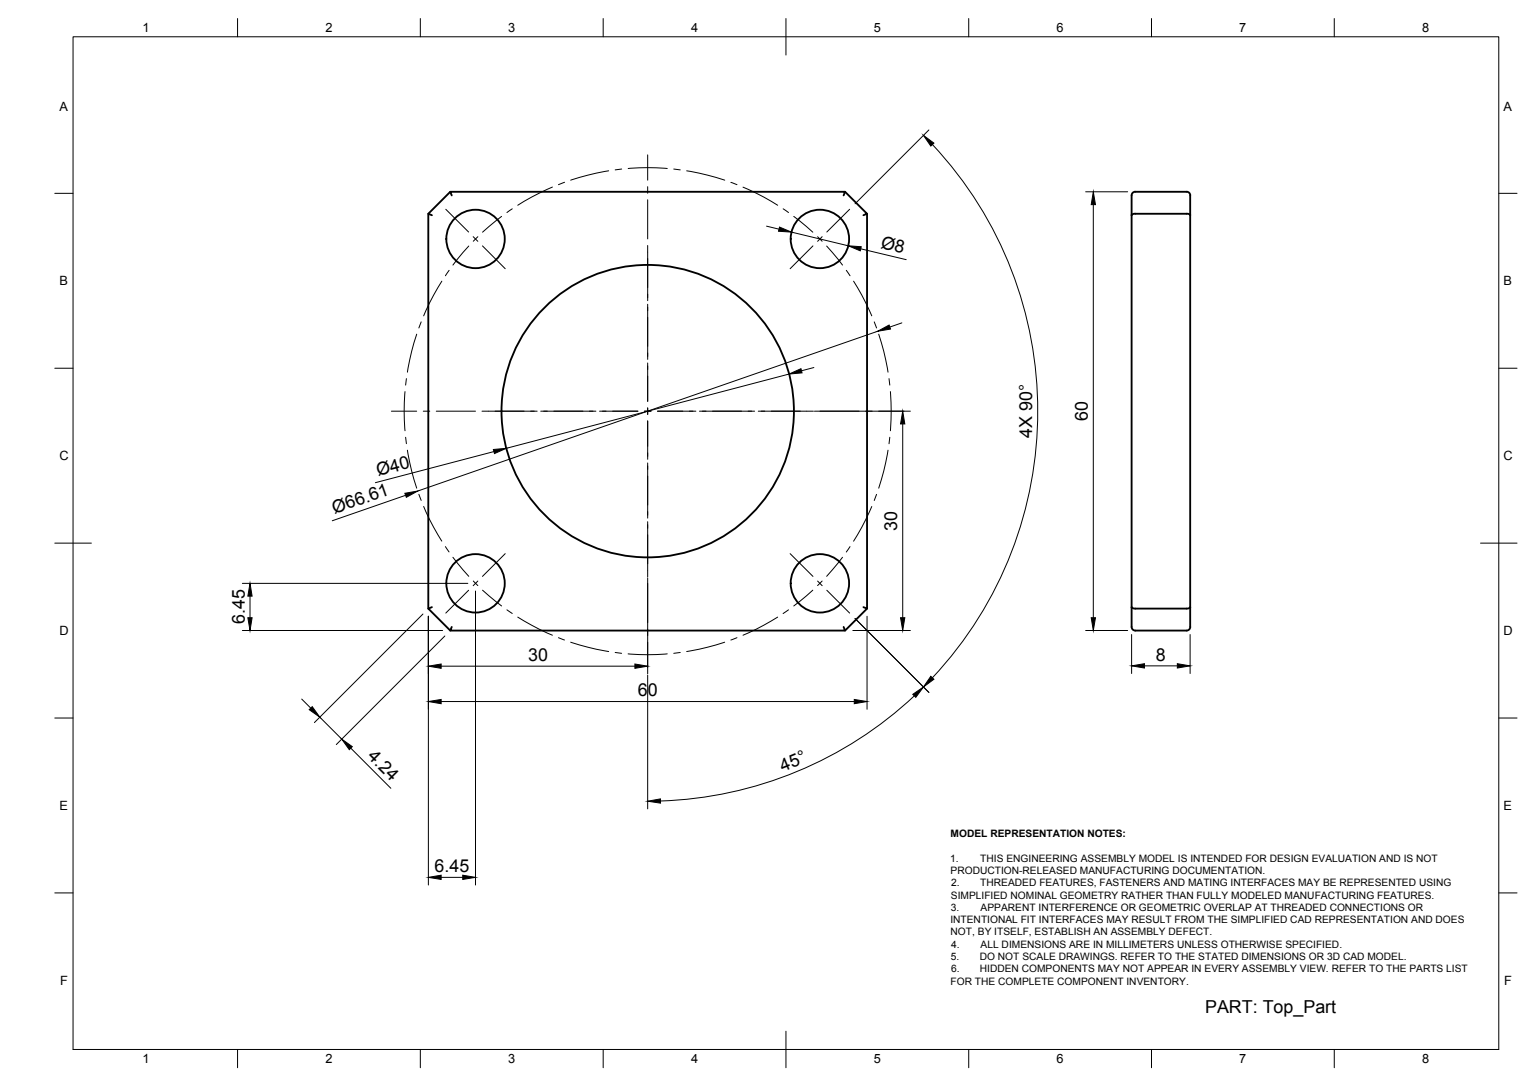
ISO-10303-21;
HEADER;
/* Generated by software containing ST-Developer
 * from STEP Tools, Inc. (www.steptools.com) 
 */

FILE_DESCRIPTION(
/* description */ (''),
/* implementation_level */ '2;1');

FILE_NAME(
/* name */ 'Top_Part.step',
/* time_stamp */ '2026-10-05T14:32:37-07:00',
/* author */ (''),
/* organization */ (''),
/* preprocessor_version */ 'ST-DEVELOPER v20.2',
/* originating_system */ 'Autodesk Translation Framework v15.15.0.0',
/* authorisation */ '');

FILE_SCHEMA (('AUTOMOTIVE_DESIGN { 1 0 10303 214 3 1 1 }'));
ENDSEC;

DATA;
#10=MECHANICAL_DESIGN_GEOMETRIC_PRESENTATION_REPRESENTATION('',(#494),#74103);
#486=SHAPE_REPRESENTATION_RELATIONSHIP('SRR','None',#74128,#490);
#490=ADVANCED_BREP_SHAPE_REPRESENTATION('',(#498),#74099);
#494=STYLED_ITEM('',(#74157),#498);
#498=MANIFOLD_SOLID_BREP('Body1',#4573);
#502=TOROIDAL_SURFACE('',#4660,4.5,0.5);
#503=TOROIDAL_SURFACE('',#4667,4.5,0.5);
#504=TOROIDAL_SURFACE('',#4674,4.5,0.5);
#505=TOROIDAL_SURFACE('',#4681,20.5,0.5);
#506=TOROIDAL_SURFACE('',#4686,4.5,0.5);
#507=TOROIDAL_SURFACE('',#4716,4.5,0.5);
#508=TOROIDAL_SURFACE('',#4718,4.5,0.5);
#509=TOROIDAL_SURFACE('',#4720,4.5,0.5);
#510=TOROIDAL_SURFACE('',#4722,20.5,0.5);
#511=TOROIDAL_SURFACE('',#4724,4.5,0.5);
#526=ELLIPSE('',#4635,0.541196100146199,0.5);
#527=ELLIPSE('',#4636,0.541196100146197,0.5);
#528=ELLIPSE('',#4638,0.541196100146197,0.5);
#529=ELLIPSE('',#4640,0.541196100146199,0.5);
#530=ELLIPSE('',#4642,0.541196100146199,0.5);
#531=ELLIPSE('',#4643,0.541196100146197,0.5);
#532=ELLIPSE('',#4645,0.541196100146197,0.5);
#533=ELLIPSE('',#4648,0.541196100146199,0.5);
#534=ELLIPSE('',#4694,0.541196100146197,0.5);
#535=ELLIPSE('',#4695,0.541196100146197,0.5);
#536=ELLIPSE('',#4697,0.541196100146197,0.5);
#537=ELLIPSE('',#4699,0.541196100146197,0.5);
#538=ELLIPSE('',#4701,0.541196100146197,0.5);
#539=ELLIPSE('',#4703,0.541196100146197,0.5);
#540=ELLIPSE('',#4705,0.541196100146197,0.5);
#541=ELLIPSE('',#4707,0.541196100146197,0.5);
#558=FACE_BOUND('',#800,.T.);
#559=FACE_BOUND('',#802,.T.);
#560=FACE_BOUND('',#817,.T.);
#561=FACE_BOUND('',#818,.T.);
#562=FACE_BOUND('',#819,.T.);
#563=FACE_BOUND('',#820,.T.);
#564=FACE_BOUND('',#821,.T.);
#565=FACE_BOUND('',#842,.T.);
#566=FACE_BOUND('',#843,.T.);
#567=FACE_BOUND('',#844,.T.);
#568=FACE_BOUND('',#845,.T.);
#569=FACE_BOUND('',#846,.T.);
#584=PLANE('',#4627);
#585=PLANE('',#4629);
#586=PLANE('',#4650);
#587=PLANE('',#4651);
#588=PLANE('',#4652);
#589=PLANE('',#4653);
#590=PLANE('',#4654);
#591=PLANE('',#4709);
#592=PLANE('',#4710);
#593=PLANE('',#4726);
#594=PLANE('',#4727);
#595=PLANE('',#4728);
#612=FACE_OUTER_BOUND('',#798,.T.);
#613=FACE_OUTER_BOUND('',#799,.T.);
#614=FACE_OUTER_BOUND('',#801,.T.);
#615=FACE_OUTER_BOUND('',#803,.T.);
#616=FACE_OUTER_BOUND('',#804,.T.);
#617=FACE_OUTER_BOUND('',#805,.T.);
#618=FACE_OUTER_BOUND('',#806,.T.);
#619=FACE_OUTER_BOUND('',#807,.T.);
#620=FACE_OUTER_BOUND('',#808,.T.);
#621=FACE_OUTER_BOUND('',#809,.T.);
#622=FACE_OUTER_BOUND('',#810,.T.);
#623=FACE_OUTER_BOUND('',#811,.T.);
#624=FACE_OUTER_BOUND('',#812,.T.);
#625=FACE_OUTER_BOUND('',#813,.T.);
#626=FACE_OUTER_BOUND('',#814,.T.);
#627=FACE_OUTER_BOUND('',#815,.T.);
#628=FACE_OUTER_BOUND('',#816,.T.);
#629=FACE_OUTER_BOUND('',#822,.T.);
#630=FACE_OUTER_BOUND('',#823,.T.);
#631=FACE_OUTER_BOUND('',#824,.T.);
#632=FACE_OUTER_BOUND('',#825,.T.);
#633=FACE_OUTER_BOUND('',#826,.T.);
#634=FACE_OUTER_BOUND('',#827,.T.);
#635=FACE_OUTER_BOUND('',#828,.T.);
#636=FACE_OUTER_BOUND('',#829,.T.);
#637=FACE_OUTER_BOUND('',#830,.T.);
#638=FACE_OUTER_BOUND('',#831,.T.);
#639=FACE_OUTER_BOUND('',#832,.T.);
#640=FACE_OUTER_BOUND('',#833,.T.);
#641=FACE_OUTER_BOUND('',#834,.T.);
#642=FACE_OUTER_BOUND('',#835,.T.);
#643=FACE_OUTER_BOUND('',#836,.T.);
#644=FACE_OUTER_BOUND('',#837,.T.);
#645=FACE_OUTER_BOUND('',#838,.T.);
#646=FACE_OUTER_BOUND('',#839,.T.);
#647=FACE_OUTER_BOUND('',#840,.T.);
#648=FACE_OUTER_BOUND('',#841,.T.);
#649=FACE_OUTER_BOUND('',#847,.T.);
#650=FACE_OUTER_BOUND('',#848,.T.);
#651=FACE_OUTER_BOUND('',#849,.T.);
#652=FACE_OUTER_BOUND('',#850,.T.);
#653=FACE_OUTER_BOUND('',#851,.T.);
#654=FACE_OUTER_BOUND('',#852,.T.);
#655=FACE_OUTER_BOUND('',#853,.T.);
#656=FACE_OUTER_BOUND('',#854,.T.);
#798=EDGE_LOOP('',(#2771,#2772,#2773,#2774));
#799=EDGE_LOOP('',(#2775));
#800=EDGE_LOOP('',(#2776));
#801=EDGE_LOOP('',(#2777));
#802=EDGE_LOOP('',(#2778));
#803=EDGE_LOOP('',(#2779,#2780,#2781,#2782,#2783));
#804=EDGE_LOOP('',(#2784,#2785,#2786,#2787));
#805=EDGE_LOOP('',(#2788,#2789,#2790,#2791));
#806=EDGE_LOOP('',(#2792,#2793,#2794,#2795));
#807=EDGE_LOOP('',(#2796,#2797,#2798,#2799));
#808=EDGE_LOOP('',(#2800,#2801,#2802,#2803));
#809=EDGE_LOOP('',(#2804,#2805,#2806,#2807));
#810=EDGE_LOOP('',(#2808,#2809,#2810,#2811));
#811=EDGE_LOOP('',(#2812,#2813,#2814,#2815));
#812=EDGE_LOOP('',(#2816,#2817,#2818,#2819));
#813=EDGE_LOOP('',(#2820,#2821,#2822,#2823));
#814=EDGE_LOOP('',(#2824,#2825,#2826,#2827));
#815=EDGE_LOOP('',(#2828,#2829,#2830,#2831));
#816=EDGE_LOOP('',(#2832,#2833,#2834,#2835,#2836,#2837,#2838,#2839));
#817=EDGE_LOOP('',(#2840));
#818=EDGE_LOOP('',(#2841));
#819=EDGE_LOOP('',(#2842));
#820=EDGE_LOOP('',(#2843));
#821=EDGE_LOOP('',(#2844));
#822=EDGE_LOOP('',(#2845,#2846,#2847,#2848,#2849));
#823=EDGE_LOOP('',(#2850,#2851,#2852,#2853,#2854,#2855));
#824=EDGE_LOOP('',(#2856,#2857,#2858,#2859,#2860));
#825=EDGE_LOOP('',(#2861,#2862,#2863,#2864,#2865,#2866));
#826=EDGE_LOOP('',(#2867,#2868,#2869,#2870,#2871));
#827=EDGE_LOOP('',(#2872,#2873,#2874,#2875,#2876,#2877));
#828=EDGE_LOOP('',(#2878,#2879,#2880,#2881,#2882));
#829=EDGE_LOOP('',(#2883,#2884,#2885,#2886,#2887));
#830=EDGE_LOOP('',(#2888,#2889,#2890,#2891,#2892));
#831=EDGE_LOOP('',(#2893,#2894,#2895,#2896,#2897,#2898));
#832=EDGE_LOOP('',(#2899,#2900,#2901,#2902));
#833=EDGE_LOOP('',(#2903,#2904,#2905,#2906));
#834=EDGE_LOOP('',(#2907,#2908,#2909,#2910));
#835=EDGE_LOOP('',(#2911,#2912,#2913,#2914));
#836=EDGE_LOOP('',(#2915,#2916,#2917,#2918));
#837=EDGE_LOOP('',(#2919,#2920,#2921,#2922));
#838=EDGE_LOOP('',(#2923,#2924,#2925,#2926));
#839=EDGE_LOOP('',(#2927,#2928,#2929,#2930));
#840=EDGE_LOOP('',(#2931,#2932,#2933,#2934));
#841=EDGE_LOOP('',(#2935,#2936,#2937,#2938,#2939,#2940,#2941,#2942));
#842=EDGE_LOOP('',(#2943));
#843=EDGE_LOOP('',(#2944));
#844=EDGE_LOOP('',(#2945));
#845=EDGE_LOOP('',(#2946));
#846=EDGE_LOOP('',(#2947));
#847=EDGE_LOOP('',(#2948,#2949,#2950,#2951,#2952));
#848=EDGE_LOOP('',(#2953,#2954,#2955,#2956,#2957));
#849=EDGE_LOOP('',(#2958,#2959,#2960,#2961,#2962));
#850=EDGE_LOOP('',(#2963,#2964,#2965,#2966,#2967));
#851=EDGE_LOOP('',(#2968,#2969,#2970,#2971,#2972));
#852=EDGE_LOOP('',(#2973,#2974,#2975,#2976));
#853=EDGE_LOOP('',(#2977,#2978,#2979,#2980));
#854=EDGE_LOOP('',(#2981,#2982,#2983,#2984));
#1010=LINE('',#5781,#1188);
#1011=LINE('',#5794,#1189);
#1012=LINE('',#5798,#1190);
#1013=LINE('',#5802,#1191);
#1014=LINE('',#5806,#1192);
#1015=LINE('',#5809,#1193);
#1016=LINE('',#5812,#1194);
#1017=LINE('',#5815,#1195);
#1018=LINE('',#5819,#1196);
#1019=LINE('',#5823,#1197);
#1020=LINE('',#5827,#1198);
#1021=LINE('',#5829,#1199);
#1022=LINE('',#5832,#1200);
#1023=LINE('',#5833,#1201);
#1024=LINE('',#5836,#1202);
#1025=LINE('',#5838,#1203);
#1026=LINE('',#5841,#1204);
#1027=LINE('',#5842,#1205);
#1028=LINE('',#5845,#1206);
#1029=LINE('',#5847,#1207);
#1030=LINE('',#5848,#1208);
#1031=LINE('',#5851,#1209);
#1032=LINE('',#5852,#1210);
#1033=LINE('',#5855,#1211);
#1034=LINE('',#5856,#1212);
#1035=LINE('',#5859,#1213);
#1036=LINE('',#5860,#1214);
#1037=LINE('',#5880,#1215);
#1038=LINE('',#5892,#1216);
#1039=LINE('',#5904,#1217);
#1040=LINE('',#5912,#1218);
#1041=LINE('',#5924,#1219);
#1042=LINE('',#5931,#1220);
#1043=LINE('',#5934,#1221);
#1044=LINE('',#5938,#1222);
#1045=LINE('',#5941,#1223);
#1046=LINE('',#5944,#1224);
#1047=LINE('',#5947,#1225);
#1048=LINE('',#5950,#1226);
#1049=LINE('',#5952,#1227);
#1050=LINE('',#5955,#1228);
#1051=LINE('',#5959,#1229);
#1052=LINE('',#5963,#1230);
#1053=LINE('',#5966,#1231);
#1054=LINE('',#5968,#1232);
#1055=LINE('',#5991,#1233);
#1056=LINE('',#5993,#1234);
#1188=VECTOR('',#4955,20.5);
#1189=VECTOR('',#4972,20.);
#1190=VECTOR('',#4975,10.);
#1191=VECTOR('',#4978,10.);
#1192=VECTOR('',#4983,10.);
#1193=VECTOR('',#4986,9.99999999999999);
#1194=VECTOR('',#4989,10.);
#1195=VECTOR('',#4992,10.);
#1196=VECTOR('',#4995,10.);
#1197=VECTOR('',#4998,10.);
#1198=VECTOR('',#5003,9.99999999999999);
#1199=VECTOR('',#5004,10.);
#1200=VECTOR('',#5009,10.);
#1201=VECTOR('',#5010,9.99999999999999);
#1202=VECTOR('',#5013,10.);
#1203=VECTOR('',#5014,10.);
#1204=VECTOR('',#5019,9.99999999999999);
#1205=VECTOR('',#5020,10.);
#1206=VECTOR('',#5023,10.);
#1207=VECTOR('',#5024,9.99999999999999);
#1208=VECTOR('',#5025,10.);
#1209=VECTOR('',#5028,10.);
#1210=VECTOR('',#5029,10.);
#1211=VECTOR('',#5032,10.);
#1212=VECTOR('',#5033,9.99999999999999);
#1213=VECTOR('',#5036,10.);
#1214=VECTOR('',#5037,10.);
#1215=VECTOR('',#5060,4.);
#1216=VECTOR('',#5075,4.);
#1217=VECTOR('',#5090,4.);
#1218=VECTOR('',#5101,20.);
#1219=VECTOR('',#5116,4.);
#1220=VECTOR('',#5123,10.);
#1221=VECTOR('',#5126,10.);
#1222=VECTOR('',#5131,10.);
#1223=VECTOR('',#5134,9.99999999999999);
#1224=VECTOR('',#5137,10.);
#1225=VECTOR('',#5140,10.);
#1226=VECTOR('',#5143,10.);
#1227=VECTOR('',#5146,9.99999999999999);
#1228=VECTOR('',#5149,10.);
#1229=VECTOR('',#5154,10.);
#1230=VECTOR('',#5159,10.);
#1231=VECTOR('',#5164,10.);
#1232=VECTOR('',#5167,10.);
#1233=VECTOR('',#5202,10.);
#1234=VECTOR('',#5205,10.);
#1366=CIRCLE('',#4625,20.5);
#1367=CIRCLE('',#4626,20.5);
#1368=CIRCLE('',#4628,20.);
#1369=CIRCLE('',#4630,20.);
#1370=CIRCLE('',#4632,20.);
#1371=CIRCLE('',#4633,20.);
#1372=CIRCLE('',#4655,4.5);
#1373=CIRCLE('',#4656,4.5);
#1374=CIRCLE('',#4657,4.5);
#1375=CIRCLE('',#4658,20.5);
#1376=CIRCLE('',#4659,4.5);
#1377=CIRCLE('',#4661,4.);
#1378=CIRCLE('',#4662,0.5);
#1379=CIRCLE('',#4663,4.);
#1380=CIRCLE('',#4665,4.);
#1381=CIRCLE('',#4666,4.);
#1382=CIRCLE('',#4668,4.);
#1383=CIRCLE('',#4669,0.5);
#1384=CIRCLE('',#4670,4.);
#1385=CIRCLE('',#4672,4.);
#1386=CIRCLE('',#4673,4.);
#1387=CIRCLE('',#4675,4.);
#1388=CIRCLE('',#4676,0.5);
#1389=CIRCLE('',#4677,4.);
#1390=CIRCLE('',#4679,4.);
#1391=CIRCLE('',#4680,4.);
#1392=CIRCLE('',#4682,0.5);
#1393=CIRCLE('',#4684,20.);
#1394=CIRCLE('',#4685,20.);
#1395=CIRCLE('',#4687,4.);
#1396=CIRCLE('',#4688,0.5);
#1397=CIRCLE('',#4689,4.);
#1398=CIRCLE('',#4691,4.);
#1399=CIRCLE('',#4692,4.);
#1400=CIRCLE('',#4711,4.5);
#1401=CIRCLE('',#4712,4.5);
#1402=CIRCLE('',#4713,4.5);
#1403=CIRCLE('',#4714,20.5);
#1404=CIRCLE('',#4715,4.5);
#1405=CIRCLE('',#4717,0.5);
#1406=CIRCLE('',#4719,0.5);
#1407=CIRCLE('',#4721,0.5);
#1408=CIRCLE('',#4723,0.5);
#1409=CIRCLE('',#4725,0.5);
#1461=VERTEX_POINT('',#5778);
#1462=VERTEX_POINT('',#5780);
#1463=VERTEX_POINT('',#5784);
#1464=VERTEX_POINT('',#5787);
#1465=VERTEX_POINT('',#5790);
#1466=VERTEX_POINT('',#5791);
#1467=VERTEX_POINT('',#5796);
#1468=VERTEX_POINT('',#5797);
#1469=VERTEX_POINT('',#5799);
#1470=VERTEX_POINT('',#5801);
#1471=VERTEX_POINT('',#5805);
#1472=VERTEX_POINT('',#5807);
#1473=VERTEX_POINT('',#5811);
#1474=VERTEX_POINT('',#5813);
#1475=VERTEX_POINT('',#5817);
#1476=VERTEX_POINT('',#5818);
#1477=VERTEX_POINT('',#5820);
#1478=VERTEX_POINT('',#5822);
#1479=VERTEX_POINT('',#5826);
#1480=VERTEX_POINT('',#5828);
#1481=VERTEX_POINT('',#5835);
#1482=VERTEX_POINT('',#5837);
#1483=VERTEX_POINT('',#5844);
#1484=VERTEX_POINT('',#5846);
#1485=VERTEX_POINT('',#5850);
#1486=VERTEX_POINT('',#5854);
#1487=VERTEX_POINT('',#5858);
#1488=VERTEX_POINT('',#5862);
#1489=VERTEX_POINT('',#5864);
#1490=VERTEX_POINT('',#5866);
#1491=VERTEX_POINT('',#5868);
#1492=VERTEX_POINT('',#5870);
#1493=VERTEX_POINT('',#5873);
#1494=VERTEX_POINT('',#5874);
#1495=VERTEX_POINT('',#5879);
#1496=VERTEX_POINT('',#5881);
#1497=VERTEX_POINT('',#5885);
#1498=VERTEX_POINT('',#5886);
#1499=VERTEX_POINT('',#5891);
#1500=VERTEX_POINT('',#5893);
#1501=VERTEX_POINT('',#5897);
#1502=VERTEX_POINT('',#5898);
#1503=VERTEX_POINT('',#5903);
#1504=VERTEX_POINT('',#5905);
#1505=VERTEX_POINT('',#5911);
#1506=VERTEX_POINT('',#5913);
#1507=VERTEX_POINT('',#5917);
#1508=VERTEX_POINT('',#5918);
#1509=VERTEX_POINT('',#5923);
#1510=VERTEX_POINT('',#5925);
#1511=VERTEX_POINT('',#5929);
#1512=VERTEX_POINT('',#5930);
#1513=VERTEX_POINT('',#5932);
#1514=VERTEX_POINT('',#5937);
#1515=VERTEX_POINT('',#5939);
#1516=VERTEX_POINT('',#5943);
#1517=VERTEX_POINT('',#5945);
#1518=VERTEX_POINT('',#5949);
#1519=VERTEX_POINT('',#5954);
#1520=VERTEX_POINT('',#5958);
#1521=VERTEX_POINT('',#5962);
#1522=VERTEX_POINT('',#5970);
#1523=VERTEX_POINT('',#5972);
#1524=VERTEX_POINT('',#5974);
#1525=VERTEX_POINT('',#5976);
#1526=VERTEX_POINT('',#5978);
#2029=EDGE_CURVE('',#1461,#1461,#1366,.T.);
#2030=EDGE_CURVE('',#1461,#1462,#1010,.T.);
#2031=EDGE_CURVE('',#1462,#1462,#1367,.T.);
#2032=EDGE_CURVE('',#1463,#1463,#1368,.T.);
#2033=EDGE_CURVE('',#1464,#1464,#1369,.T.);
#2034=EDGE_CURVE('',#1465,#1466,#1370,.T.);
#2035=EDGE_CURVE('',#1466,#1465,#1371,.T.);
#2036=EDGE_CURVE('',#1466,#1464,#1011,.T.);
#2037=EDGE_CURVE('',#1467,#1468,#1012,.T.);
#2038=EDGE_CURVE('',#1468,#1469,#526,.T.);
#2039=EDGE_CURVE('',#1469,#1470,#1013,.T.);
#2040=EDGE_CURVE('',#1467,#1470,#527,.T.);
#2041=EDGE_CURVE('',#1468,#1471,#1014,.T.);
#2042=EDGE_CURVE('',#1471,#1472,#528,.T.);
#2043=EDGE_CURVE('',#1472,#1469,#1015,.T.);
#2044=EDGE_CURVE('',#1471,#1473,#1016,.T.);
#2045=EDGE_CURVE('',#1473,#1474,#529,.T.);
#2046=EDGE_CURVE('',#1474,#1472,#1017,.T.);
#2047=EDGE_CURVE('',#1475,#1476,#1018,.T.);
#2048=EDGE_CURVE('',#1476,#1477,#530,.T.);
#2049=EDGE_CURVE('',#1477,#1478,#1019,.T.);
#2050=EDGE_CURVE('',#1478,#1475,#531,.T.);
#2051=EDGE_CURVE('',#1479,#1477,#1020,.T.);
#2052=EDGE_CURVE('',#1476,#1480,#1021,.T.);
#2053=EDGE_CURVE('',#1480,#1479,#532,.T.);
#2054=EDGE_CURVE('',#1473,#1475,#1022,.T.);
#2055=EDGE_CURVE('',#1478,#1474,#1023,.T.);
#2056=EDGE_CURVE('',#1481,#1479,#1024,.T.);
#2057=EDGE_CURVE('',#1480,#1482,#1025,.T.);
#2058=EDGE_CURVE('',#1482,#1481,#533,.T.);
#2059=EDGE_CURVE('',#1470,#1481,#1026,.T.);
#2060=EDGE_CURVE('',#1482,#1467,#1027,.T.);
#2061=EDGE_CURVE('',#1472,#1483,#1028,.T.);
#2062=EDGE_CURVE('',#1484,#1483,#1029,.T.);
#2063=EDGE_CURVE('',#1469,#1484,#1030,.T.);
#2064=EDGE_CURVE('',#1474,#1485,#1031,.T.);
#2065=EDGE_CURVE('',#1483,#1485,#1032,.T.);
#2066=EDGE_CURVE('',#1478,#1486,#1033,.T.);
#2067=EDGE_CURVE('',#1485,#1486,#1034,.T.);
#2068=EDGE_CURVE('',#1477,#1487,#1035,.T.);
#2069=EDGE_CURVE('',#1486,#1487,#1036,.T.);
#2070=EDGE_CURVE('',#1488,#1488,#1372,.T.);
#2071=EDGE_CURVE('',#1489,#1489,#1373,.T.);
#2072=EDGE_CURVE('',#1490,#1490,#1374,.T.);
#2073=EDGE_CURVE('',#1491,#1491,#1375,.T.);
#2074=EDGE_CURVE('',#1492,#1492,#1376,.T.);
#2075=EDGE_CURVE('',#1493,#1494,#1377,.T.);
#2076=EDGE_CURVE('',#1494,#1488,#1378,.T.);
#2077=EDGE_CURVE('',#1494,#1493,#1379,.T.);
#2078=EDGE_CURVE('',#1493,#1495,#1037,.T.);
#2079=EDGE_CURVE('',#1496,#1495,#1380,.T.);
#2080=EDGE_CURVE('',#1495,#1496,#1381,.T.);
#2081=EDGE_CURVE('',#1497,#1498,#1382,.T.);
#2082=EDGE_CURVE('',#1498,#1492,#1383,.T.);
#2083=EDGE_CURVE('',#1498,#1497,#1384,.T.);
#2084=EDGE_CURVE('',#1497,#1499,#1038,.T.);
#2085=EDGE_CURVE('',#1500,#1499,#1385,.T.);
#2086=EDGE_CURVE('',#1499,#1500,#1386,.T.);
#2087=EDGE_CURVE('',#1501,#1502,#1387,.T.);
#2088=EDGE_CURVE('',#1502,#1489,#1388,.T.);
#2089=EDGE_CURVE('',#1502,#1501,#1389,.T.);
#2090=EDGE_CURVE('',#1501,#1503,#1039,.T.);
#2091=EDGE_CURVE('',#1504,#1503,#1390,.T.);
#2092=EDGE_CURVE('',#1503,#1504,#1391,.T.);
#2093=EDGE_CURVE('',#1465,#1491,#1392,.T.);
#2094=EDGE_CURVE('',#1463,#1505,#1040,.T.);
#2095=EDGE_CURVE('',#1506,#1505,#1393,.T.);
#2096=EDGE_CURVE('',#1505,#1506,#1394,.T.);
#2097=EDGE_CURVE('',#1507,#1508,#1395,.T.);
#2098=EDGE_CURVE('',#1508,#1490,#1396,.T.);
#2099=EDGE_CURVE('',#1508,#1507,#1397,.T.);
#2100=EDGE_CURVE('',#1507,#1509,#1041,.T.);
#2101=EDGE_CURVE('',#1510,#1509,#1398,.T.);
#2102=EDGE_CURVE('',#1509,#1510,#1399,.T.);
#2103=EDGE_CURVE('',#1511,#1512,#1042,.T.);
#2104=EDGE_CURVE('',#1512,#1513,#534,.T.);
#2105=EDGE_CURVE('',#1513,#1484,#1043,.T.);
#2106=EDGE_CURVE('',#1511,#1484,#535,.T.);
#2107=EDGE_CURVE('',#1512,#1514,#1044,.T.);
#2108=EDGE_CURVE('',#1514,#1515,#536,.T.);
#2109=EDGE_CURVE('',#1515,#1513,#1045,.T.);
#2110=EDGE_CURVE('',#1514,#1516,#1046,.T.);
#2111=EDGE_CURVE('',#1516,#1517,#537,.T.);
#2112=EDGE_CURVE('',#1517,#1515,#1047,.T.);
#2113=EDGE_CURVE('',#1516,#1518,#1048,.T.);
#2114=EDGE_CURVE('',#1518,#1487,#538,.T.);
#2115=EDGE_CURVE('',#1487,#1517,#1049,.T.);
#2116=EDGE_CURVE('',#1518,#1519,#1050,.T.);
#2117=EDGE_CURVE('',#1519,#1486,#539,.T.);
#2118=EDGE_CURVE('',#1519,#1520,#1051,.T.);
#2119=EDGE_CURVE('',#1520,#1485,#540,.T.);
#2120=EDGE_CURVE('',#1520,#1521,#1052,.T.);
#2121=EDGE_CURVE('',#1521,#1483,#541,.T.);
#2122=EDGE_CURVE('',#1521,#1511,#1053,.T.);
#2123=EDGE_CURVE('',#1470,#1513,#1054,.T.);
#2124=EDGE_CURVE('',#1522,#1522,#1400,.T.);
#2125=EDGE_CURVE('',#1523,#1523,#1401,.T.);
#2126=EDGE_CURVE('',#1524,#1524,#1402,.T.);
#2127=EDGE_CURVE('',#1525,#1525,#1403,.T.);
#2128=EDGE_CURVE('',#1526,#1526,#1404,.T.);
#2129=EDGE_CURVE('',#1522,#1496,#1405,.T.);
#2130=EDGE_CURVE('',#1526,#1500,#1406,.T.);
#2131=EDGE_CURVE('',#1523,#1504,#1407,.T.);
#2132=EDGE_CURVE('',#1525,#1506,#1408,.T.);
#2133=EDGE_CURVE('',#1524,#1510,#1409,.T.);
#2134=EDGE_CURVE('',#1481,#1515,#1055,.T.);
#2135=EDGE_CURVE('',#1479,#1517,#1056,.T.);
#2771=ORIENTED_EDGE('',*,*,#2029,.F.);
#2772=ORIENTED_EDGE('',*,*,#2030,.T.);
#2773=ORIENTED_EDGE('',*,*,#2031,.T.);
#2774=ORIENTED_EDGE('',*,*,#2030,.F.);
#2775=ORIENTED_EDGE('',*,*,#2031,.F.);
#2776=ORIENTED_EDGE('',*,*,#2032,.F.);
#2777=ORIENTED_EDGE('',*,*,#2029,.T.);
#2778=ORIENTED_EDGE('',*,*,#2033,.F.);
#2779=ORIENTED_EDGE('',*,*,#2034,.F.);
#2780=ORIENTED_EDGE('',*,*,#2035,.F.);
#2781=ORIENTED_EDGE('',*,*,#2036,.T.);
#2782=ORIENTED_EDGE('',*,*,#2033,.T.);
#2783=ORIENTED_EDGE('',*,*,#2036,.F.);
#2784=ORIENTED_EDGE('',*,*,#2037,.T.);
#2785=ORIENTED_EDGE('',*,*,#2038,.T.);
#2786=ORIENTED_EDGE('',*,*,#2039,.T.);
#2787=ORIENTED_EDGE('',*,*,#2040,.F.);
#2788=ORIENTED_EDGE('',*,*,#2041,.T.);
#2789=ORIENTED_EDGE('',*,*,#2042,.T.);
#2790=ORIENTED_EDGE('',*,*,#2043,.T.);
#2791=ORIENTED_EDGE('',*,*,#2038,.F.);
#2792=ORIENTED_EDGE('',*,*,#2044,.T.);
#2793=ORIENTED_EDGE('',*,*,#2045,.T.);
#2794=ORIENTED_EDGE('',*,*,#2046,.T.);
#2795=ORIENTED_EDGE('',*,*,#2042,.F.);
#2796=ORIENTED_EDGE('',*,*,#2047,.T.);
#2797=ORIENTED_EDGE('',*,*,#2048,.T.);
#2798=ORIENTED_EDGE('',*,*,#2049,.T.);
#2799=ORIENTED_EDGE('',*,*,#2050,.T.);
#2800=ORIENTED_EDGE('',*,*,#2051,.T.);
#2801=ORIENTED_EDGE('',*,*,#2048,.F.);
#2802=ORIENTED_EDGE('',*,*,#2052,.T.);
#2803=ORIENTED_EDGE('',*,*,#2053,.T.);
#2804=ORIENTED_EDGE('',*,*,#2054,.T.);
#2805=ORIENTED_EDGE('',*,*,#2050,.F.);
#2806=ORIENTED_EDGE('',*,*,#2055,.T.);
#2807=ORIENTED_EDGE('',*,*,#2045,.F.);
#2808=ORIENTED_EDGE('',*,*,#2056,.T.);
#2809=ORIENTED_EDGE('',*,*,#2053,.F.);
#2810=ORIENTED_EDGE('',*,*,#2057,.T.);
#2811=ORIENTED_EDGE('',*,*,#2058,.T.);
#2812=ORIENTED_EDGE('',*,*,#2059,.T.);
#2813=ORIENTED_EDGE('',*,*,#2058,.F.);
#2814=ORIENTED_EDGE('',*,*,#2060,.T.);
#2815=ORIENTED_EDGE('',*,*,#2040,.T.);
#2816=ORIENTED_EDGE('',*,*,#2043,.F.);
#2817=ORIENTED_EDGE('',*,*,#2061,.T.);
#2818=ORIENTED_EDGE('',*,*,#2062,.F.);
#2819=ORIENTED_EDGE('',*,*,#2063,.F.);
#2820=ORIENTED_EDGE('',*,*,#2046,.F.);
#2821=ORIENTED_EDGE('',*,*,#2064,.T.);
#2822=ORIENTED_EDGE('',*,*,#2065,.F.);
#2823=ORIENTED_EDGE('',*,*,#2061,.F.);
#2824=ORIENTED_EDGE('',*,*,#2055,.F.);
#2825=ORIENTED_EDGE('',*,*,#2066,.T.);
#2826=ORIENTED_EDGE('',*,*,#2067,.F.);
#2827=ORIENTED_EDGE('',*,*,#2064,.F.);
#2828=ORIENTED_EDGE('',*,*,#2049,.F.);
#2829=ORIENTED_EDGE('',*,*,#2068,.T.);
#2830=ORIENTED_EDGE('',*,*,#2069,.F.);
#2831=ORIENTED_EDGE('',*,*,#2066,.F.);
#2832=ORIENTED_EDGE('',*,*,#2047,.F.);
#2833=ORIENTED_EDGE('',*,*,#2054,.F.);
#2834=ORIENTED_EDGE('',*,*,#2044,.F.);
#2835=ORIENTED_EDGE('',*,*,#2041,.F.);
#2836=ORIENTED_EDGE('',*,*,#2037,.F.);
#2837=ORIENTED_EDGE('',*,*,#2060,.F.);
#2838=ORIENTED_EDGE('',*,*,#2057,.F.);
#2839=ORIENTED_EDGE('',*,*,#2052,.F.);
#2840=ORIENTED_EDGE('',*,*,#2070,.F.);
#2841=ORIENTED_EDGE('',*,*,#2071,.F.);
#2842=ORIENTED_EDGE('',*,*,#2072,.F.);
#2843=ORIENTED_EDGE('',*,*,#2073,.F.);
#2844=ORIENTED_EDGE('',*,*,#2074,.F.);
#2845=ORIENTED_EDGE('',*,*,#2075,.T.);
#2846=ORIENTED_EDGE('',*,*,#2076,.T.);
#2847=ORIENTED_EDGE('',*,*,#2070,.T.);
#2848=ORIENTED_EDGE('',*,*,#2076,.F.);
#2849=ORIENTED_EDGE('',*,*,#2077,.T.);
#2850=ORIENTED_EDGE('',*,*,#2075,.F.);
#2851=ORIENTED_EDGE('',*,*,#2078,.T.);
#2852=ORIENTED_EDGE('',*,*,#2079,.F.);
#2853=ORIENTED_EDGE('',*,*,#2080,.F.);
#2854=ORIENTED_EDGE('',*,*,#2078,.F.);
#2855=ORIENTED_EDGE('',*,*,#2077,.F.);
#2856=ORIENTED_EDGE('',*,*,#2081,.T.);
#2857=ORIENTED_EDGE('',*,*,#2082,.T.);
#2858=ORIENTED_EDGE('',*,*,#2074,.T.);
#2859=ORIENTED_EDGE('',*,*,#2082,.F.);
#2860=ORIENTED_EDGE('',*,*,#2083,.T.);
#2861=ORIENTED_EDGE('',*,*,#2081,.F.);
#2862=ORIENTED_EDGE('',*,*,#2084,.T.);
#2863=ORIENTED_EDGE('',*,*,#2085,.F.);
#2864=ORIENTED_EDGE('',*,*,#2086,.F.);
#2865=ORIENTED_EDGE('',*,*,#2084,.F.);
#2866=ORIENTED_EDGE('',*,*,#2083,.F.);
#2867=ORIENTED_EDGE('',*,*,#2087,.T.);
#2868=ORIENTED_EDGE('',*,*,#2088,.T.);
#2869=ORIENTED_EDGE('',*,*,#2071,.T.);
#2870=ORIENTED_EDGE('',*,*,#2088,.F.);
#2871=ORIENTED_EDGE('',*,*,#2089,.T.);
#2872=ORIENTED_EDGE('',*,*,#2087,.F.);
#2873=ORIENTED_EDGE('',*,*,#2090,.T.);
#2874=ORIENTED_EDGE('',*,*,#2091,.F.);
#2875=ORIENTED_EDGE('',*,*,#2092,.F.);
#2876=ORIENTED_EDGE('',*,*,#2090,.F.);
#2877=ORIENTED_EDGE('',*,*,#2089,.F.);
#2878=ORIENTED_EDGE('',*,*,#2034,.T.);
#2879=ORIENTED_EDGE('',*,*,#2035,.T.);
#2880=ORIENTED_EDGE('',*,*,#2093,.T.);
#2881=ORIENTED_EDGE('',*,*,#2073,.T.);
#2882=ORIENTED_EDGE('',*,*,#2093,.F.);
#2883=ORIENTED_EDGE('',*,*,#2032,.T.);
#2884=ORIENTED_EDGE('',*,*,#2094,.T.);
#2885=ORIENTED_EDGE('',*,*,#2095,.F.);
#2886=ORIENTED_EDGE('',*,*,#2096,.F.);
#2887=ORIENTED_EDGE('',*,*,#2094,.F.);
#2888=ORIENTED_EDGE('',*,*,#2097,.T.);
#2889=ORIENTED_EDGE('',*,*,#2098,.T.);
#2890=ORIENTED_EDGE('',*,*,#2072,.T.);
#2891=ORIENTED_EDGE('',*,*,#2098,.F.);
#2892=ORIENTED_EDGE('',*,*,#2099,.T.);
#2893=ORIENTED_EDGE('',*,*,#2097,.F.);
#2894=ORIENTED_EDGE('',*,*,#2100,.T.);
#2895=ORIENTED_EDGE('',*,*,#2101,.F.);
#2896=ORIENTED_EDGE('',*,*,#2102,.F.);
#2897=ORIENTED_EDGE('',*,*,#2100,.F.);
#2898=ORIENTED_EDGE('',*,*,#2099,.F.);
#2899=ORIENTED_EDGE('',*,*,#2103,.T.);
#2900=ORIENTED_EDGE('',*,*,#2104,.T.);
#2901=ORIENTED_EDGE('',*,*,#2105,.T.);
#2902=ORIENTED_EDGE('',*,*,#2106,.F.);
#2903=ORIENTED_EDGE('',*,*,#2107,.T.);
#2904=ORIENTED_EDGE('',*,*,#2108,.T.);
#2905=ORIENTED_EDGE('',*,*,#2109,.T.);
#2906=ORIENTED_EDGE('',*,*,#2104,.F.);
#2907=ORIENTED_EDGE('',*,*,#2110,.T.);
#2908=ORIENTED_EDGE('',*,*,#2111,.T.);
#2909=ORIENTED_EDGE('',*,*,#2112,.T.);
#2910=ORIENTED_EDGE('',*,*,#2108,.F.);
#2911=ORIENTED_EDGE('',*,*,#2113,.T.);
#2912=ORIENTED_EDGE('',*,*,#2114,.T.);
#2913=ORIENTED_EDGE('',*,*,#2115,.T.);
#2914=ORIENTED_EDGE('',*,*,#2111,.F.);
#2915=ORIENTED_EDGE('',*,*,#2116,.T.);
#2916=ORIENTED_EDGE('',*,*,#2117,.T.);
#2917=ORIENTED_EDGE('',*,*,#2069,.T.);
#2918=ORIENTED_EDGE('',*,*,#2114,.F.);
#2919=ORIENTED_EDGE('',*,*,#2067,.T.);
#2920=ORIENTED_EDGE('',*,*,#2117,.F.);
#2921=ORIENTED_EDGE('',*,*,#2118,.T.);
#2922=ORIENTED_EDGE('',*,*,#2119,.T.);
#2923=ORIENTED_EDGE('',*,*,#2065,.T.);
#2924=ORIENTED_EDGE('',*,*,#2119,.F.);
#2925=ORIENTED_EDGE('',*,*,#2120,.T.);
#2926=ORIENTED_EDGE('',*,*,#2121,.T.);
#2927=ORIENTED_EDGE('',*,*,#2062,.T.);
#2928=ORIENTED_EDGE('',*,*,#2121,.F.);
#2929=ORIENTED_EDGE('',*,*,#2122,.T.);
#2930=ORIENTED_EDGE('',*,*,#2106,.T.);
#2931=ORIENTED_EDGE('',*,*,#2039,.F.);
#2932=ORIENTED_EDGE('',*,*,#2063,.T.);
#2933=ORIENTED_EDGE('',*,*,#2105,.F.);
#2934=ORIENTED_EDGE('',*,*,#2123,.F.);
#2935=ORIENTED_EDGE('',*,*,#2103,.F.);
#2936=ORIENTED_EDGE('',*,*,#2122,.F.);
#2937=ORIENTED_EDGE('',*,*,#2120,.F.);
#2938=ORIENTED_EDGE('',*,*,#2118,.F.);
#2939=ORIENTED_EDGE('',*,*,#2116,.F.);
#2940=ORIENTED_EDGE('',*,*,#2113,.F.);
#2941=ORIENTED_EDGE('',*,*,#2110,.F.);
#2942=ORIENTED_EDGE('',*,*,#2107,.F.);
#2943=ORIENTED_EDGE('',*,*,#2124,.F.);
#2944=ORIENTED_EDGE('',*,*,#2125,.F.);
#2945=ORIENTED_EDGE('',*,*,#2126,.F.);
#2946=ORIENTED_EDGE('',*,*,#2127,.F.);
#2947=ORIENTED_EDGE('',*,*,#2128,.F.);
#2948=ORIENTED_EDGE('',*,*,#2124,.T.);
#2949=ORIENTED_EDGE('',*,*,#2129,.T.);
#2950=ORIENTED_EDGE('',*,*,#2079,.T.);
#2951=ORIENTED_EDGE('',*,*,#2080,.T.);
#2952=ORIENTED_EDGE('',*,*,#2129,.F.);
#2953=ORIENTED_EDGE('',*,*,#2128,.T.);
#2954=ORIENTED_EDGE('',*,*,#2130,.T.);
#2955=ORIENTED_EDGE('',*,*,#2085,.T.);
#2956=ORIENTED_EDGE('',*,*,#2086,.T.);
#2957=ORIENTED_EDGE('',*,*,#2130,.F.);
#2958=ORIENTED_EDGE('',*,*,#2125,.T.);
#2959=ORIENTED_EDGE('',*,*,#2131,.T.);
#2960=ORIENTED_EDGE('',*,*,#2091,.T.);
#2961=ORIENTED_EDGE('',*,*,#2092,.T.);
#2962=ORIENTED_EDGE('',*,*,#2131,.F.);
#2963=ORIENTED_EDGE('',*,*,#2127,.T.);
#2964=ORIENTED_EDGE('',*,*,#2132,.T.);
#2965=ORIENTED_EDGE('',*,*,#2095,.T.);
#2966=ORIENTED_EDGE('',*,*,#2096,.T.);
#2967=ORIENTED_EDGE('',*,*,#2132,.F.);
#2968=ORIENTED_EDGE('',*,*,#2126,.T.);
#2969=ORIENTED_EDGE('',*,*,#2133,.T.);
#2970=ORIENTED_EDGE('',*,*,#2101,.T.);
#2971=ORIENTED_EDGE('',*,*,#2102,.T.);
#2972=ORIENTED_EDGE('',*,*,#2133,.F.);
#2973=ORIENTED_EDGE('',*,*,#2059,.F.);
#2974=ORIENTED_EDGE('',*,*,#2123,.T.);
#2975=ORIENTED_EDGE('',*,*,#2109,.F.);
#2976=ORIENTED_EDGE('',*,*,#2134,.F.);
#2977=ORIENTED_EDGE('',*,*,#2056,.F.);
#2978=ORIENTED_EDGE('',*,*,#2134,.T.);
#2979=ORIENTED_EDGE('',*,*,#2112,.F.);
#2980=ORIENTED_EDGE('',*,*,#2135,.F.);
#2981=ORIENTED_EDGE('',*,*,#2051,.F.);
#2982=ORIENTED_EDGE('',*,*,#2135,.T.);
#2983=ORIENTED_EDGE('',*,*,#2115,.F.);
#2984=ORIENTED_EDGE('',*,*,#2068,.F.);
#4255=CYLINDRICAL_SURFACE('',#4624,20.5);
#4256=CYLINDRICAL_SURFACE('',#4631,20.);
#4257=CYLINDRICAL_SURFACE('',#4634,0.5);
#4258=CYLINDRICAL_SURFACE('',#4637,0.5);
#4259=CYLINDRICAL_SURFACE('',#4639,0.5);
#4260=CYLINDRICAL_SURFACE('',#4641,0.5);
#4261=CYLINDRICAL_SURFACE('',#4644,0.5);
#4262=CYLINDRICAL_SURFACE('',#4646,0.5);
#4263=CYLINDRICAL_SURFACE('',#4647,0.5);
#4264=CYLINDRICAL_SURFACE('',#4649,0.5);
#4265=CYLINDRICAL_SURFACE('',#4664,4.);
#4266=CYLINDRICAL_SURFACE('',#4671,4.);
#4267=CYLINDRICAL_SURFACE('',#4678,4.);
#4268=CYLINDRICAL_SURFACE('',#4683,20.);
#4269=CYLINDRICAL_SURFACE('',#4690,4.);
#4270=CYLINDRICAL_SURFACE('',#4693,0.5);
#4271=CYLINDRICAL_SURFACE('',#4696,0.5);
#4272=CYLINDRICAL_SURFACE('',#4698,0.5);
#4273=CYLINDRICAL_SURFACE('',#4700,0.5);
#4274=CYLINDRICAL_SURFACE('',#4702,0.5);
#4275=CYLINDRICAL_SURFACE('',#4704,0.5);
#4276=CYLINDRICAL_SURFACE('',#4706,0.5);
#4277=CYLINDRICAL_SURFACE('',#4708,0.5);
#4387=ADVANCED_FACE('',(#612),#4255,.F.);
#4388=ADVANCED_FACE('',(#613,#558),#584,.F.);
#4389=ADVANCED_FACE('',(#614,#559),#585,.F.);
#4390=ADVANCED_FACE('',(#615),#4256,.F.);
#4391=ADVANCED_FACE('',(#616),#4257,.T.);
#4392=ADVANCED_FACE('',(#617),#4258,.T.);
#4393=ADVANCED_FACE('',(#618),#4259,.T.);
#4394=ADVANCED_FACE('',(#619),#4260,.T.);
#4395=ADVANCED_FACE('',(#620),#4261,.T.);
#4396=ADVANCED_FACE('',(#621),#4262,.T.);
#4397=ADVANCED_FACE('',(#622),#4263,.T.);
#4398=ADVANCED_FACE('',(#623),#4264,.T.);
#4399=ADVANCED_FACE('',(#624),#586,.T.);
#4400=ADVANCED_FACE('',(#625),#587,.T.);
#4401=ADVANCED_FACE('',(#626),#588,.T.);
#4402=ADVANCED_FACE('',(#627),#589,.T.);
#4403=ADVANCED_FACE('',(#628,#560,#561,#562,#563,#564),#590,.F.);
#4404=ADVANCED_FACE('',(#629),#502,.T.);
#4405=ADVANCED_FACE('',(#630),#4265,.F.);
#4406=ADVANCED_FACE('',(#631),#503,.T.);
#4407=ADVANCED_FACE('',(#632),#4266,.F.);
#4408=ADVANCED_FACE('',(#633),#504,.T.);
#4409=ADVANCED_FACE('',(#634),#4267,.F.);
#4410=ADVANCED_FACE('',(#635),#505,.T.);
#4411=ADVANCED_FACE('',(#636),#4268,.F.);
#4412=ADVANCED_FACE('',(#637),#506,.T.);
#4413=ADVANCED_FACE('',(#638),#4269,.F.);
#4414=ADVANCED_FACE('',(#639),#4270,.T.);
#4415=ADVANCED_FACE('',(#640),#4271,.T.);
#4416=ADVANCED_FACE('',(#641),#4272,.T.);
#4417=ADVANCED_FACE('',(#642),#4273,.T.);
#4418=ADVANCED_FACE('',(#643),#4274,.T.);
#4419=ADVANCED_FACE('',(#644),#4275,.T.);
#4420=ADVANCED_FACE('',(#645),#4276,.T.);
#4421=ADVANCED_FACE('',(#646),#4277,.T.);
#4422=ADVANCED_FACE('',(#647),#591,.T.);
#4423=ADVANCED_FACE('',(#648,#565,#566,#567,#568,#569),#592,.T.);
#4424=ADVANCED_FACE('',(#649),#507,.T.);
#4425=ADVANCED_FACE('',(#650),#508,.T.);
#4426=ADVANCED_FACE('',(#651),#509,.T.);
#4427=ADVANCED_FACE('',(#652),#510,.T.);
#4428=ADVANCED_FACE('',(#653),#511,.T.);
#4429=ADVANCED_FACE('',(#654),#593,.T.);
#4430=ADVANCED_FACE('',(#655),#594,.T.);
#4431=ADVANCED_FACE('',(#656),#595,.T.);
#4573=CLOSED_SHELL('',(#4387,#4388,#4389,#4390,#4391,#4392,#4393,#4394,
#4395,#4396,#4397,#4398,#4399,#4400,#4401,#4402,#4403,#4404,#4405,#4406,
#4407,#4408,#4409,#4410,#4411,#4412,#4413,#4414,#4415,#4416,#4417,#4418,
#4419,#4420,#4421,#4422,#4423,#4424,#4425,#4426,#4427,#4428,#4429,#4430,
#4431));
#4623=AXIS2_PLACEMENT_3D('',#5776,#4949,#4950);
#4624=AXIS2_PLACEMENT_3D('',#5777,#4951,#4952);
#4625=AXIS2_PLACEMENT_3D('',#5779,#4953,#4954);
#4626=AXIS2_PLACEMENT_3D('',#5782,#4956,#4957);
#4627=AXIS2_PLACEMENT_3D('',#5783,#4958,#4959);
#4628=AXIS2_PLACEMENT_3D('',#5785,#4960,#4961);
#4629=AXIS2_PLACEMENT_3D('',#5786,#4962,#4963);
#4630=AXIS2_PLACEMENT_3D('',#5788,#4964,#4965);
#4631=AXIS2_PLACEMENT_3D('',#5789,#4966,#4967);
#4632=AXIS2_PLACEMENT_3D('',#5792,#4968,#4969);
#4633=AXIS2_PLACEMENT_3D('',#5793,#4970,#4971);
#4634=AXIS2_PLACEMENT_3D('',#5795,#4973,#4974);
#4635=AXIS2_PLACEMENT_3D('',#5800,#4976,#4977);
#4636=AXIS2_PLACEMENT_3D('',#5803,#4979,#4980);
#4637=AXIS2_PLACEMENT_3D('',#5804,#4981,#4982);
#4638=AXIS2_PLACEMENT_3D('',#5808,#4984,#4985);
#4639=AXIS2_PLACEMENT_3D('',#5810,#4987,#4988);
#4640=AXIS2_PLACEMENT_3D('',#5814,#4990,#4991);
#4641=AXIS2_PLACEMENT_3D('',#5816,#4993,#4994);
#4642=AXIS2_PLACEMENT_3D('',#5821,#4996,#4997);
#4643=AXIS2_PLACEMENT_3D('',#5824,#4999,#5000);
#4644=AXIS2_PLACEMENT_3D('',#5825,#5001,#5002);
#4645=AXIS2_PLACEMENT_3D('',#5830,#5005,#5006);
#4646=AXIS2_PLACEMENT_3D('',#5831,#5007,#5008);
#4647=AXIS2_PLACEMENT_3D('',#5834,#5011,#5012);
#4648=AXIS2_PLACEMENT_3D('',#5839,#5015,#5016);
#4649=AXIS2_PLACEMENT_3D('',#5840,#5017,#5018);
#4650=AXIS2_PLACEMENT_3D('',#5843,#5021,#5022);
#4651=AXIS2_PLACEMENT_3D('',#5849,#5026,#5027);
#4652=AXIS2_PLACEMENT_3D('',#5853,#5030,#5031);
#4653=AXIS2_PLACEMENT_3D('',#5857,#5034,#5035);
#4654=AXIS2_PLACEMENT_3D('',#5861,#5038,#5039);
#4655=AXIS2_PLACEMENT_3D('',#5863,#5040,#5041);
#4656=AXIS2_PLACEMENT_3D('',#5865,#5042,#5043);
#4657=AXIS2_PLACEMENT_3D('',#5867,#5044,#5045);
#4658=AXIS2_PLACEMENT_3D('',#5869,#5046,#5047);
#4659=AXIS2_PLACEMENT_3D('',#5871,#5048,#5049);
#4660=AXIS2_PLACEMENT_3D('',#5872,#5050,#5051);
#4661=AXIS2_PLACEMENT_3D('',#5875,#5052,#5053);
#4662=AXIS2_PLACEMENT_3D('',#5876,#5054,#5055);
#4663=AXIS2_PLACEMENT_3D('',#5877,#5056,#5057);
#4664=AXIS2_PLACEMENT_3D('',#5878,#5058,#5059);
#4665=AXIS2_PLACEMENT_3D('',#5882,#5061,#5062);
#4666=AXIS2_PLACEMENT_3D('',#5883,#5063,#5064);
#4667=AXIS2_PLACEMENT_3D('',#5884,#5065,#5066);
#4668=AXIS2_PLACEMENT_3D('',#5887,#5067,#5068);
#4669=AXIS2_PLACEMENT_3D('',#5888,#5069,#5070);
#4670=AXIS2_PLACEMENT_3D('',#5889,#5071,#5072);
#4671=AXIS2_PLACEMENT_3D('',#5890,#5073,#5074);
#4672=AXIS2_PLACEMENT_3D('',#5894,#5076,#5077);
#4673=AXIS2_PLACEMENT_3D('',#5895,#5078,#5079);
#4674=AXIS2_PLACEMENT_3D('',#5896,#5080,#5081);
#4675=AXIS2_PLACEMENT_3D('',#5899,#5082,#5083);
#4676=AXIS2_PLACEMENT_3D('',#5900,#5084,#5085);
#4677=AXIS2_PLACEMENT_3D('',#5901,#5086,#5087);
#4678=AXIS2_PLACEMENT_3D('',#5902,#5088,#5089);
#4679=AXIS2_PLACEMENT_3D('',#5906,#5091,#5092);
#4680=AXIS2_PLACEMENT_3D('',#5907,#5093,#5094);
#4681=AXIS2_PLACEMENT_3D('',#5908,#5095,#5096);
#4682=AXIS2_PLACEMENT_3D('',#5909,#5097,#5098);
#4683=AXIS2_PLACEMENT_3D('',#5910,#5099,#5100);
#4684=AXIS2_PLACEMENT_3D('',#5914,#5102,#5103);
#4685=AXIS2_PLACEMENT_3D('',#5915,#5104,#5105);
#4686=AXIS2_PLACEMENT_3D('',#5916,#5106,#5107);
#4687=AXIS2_PLACEMENT_3D('',#5919,#5108,#5109);
#4688=AXIS2_PLACEMENT_3D('',#5920,#5110,#5111);
#4689=AXIS2_PLACEMENT_3D('',#5921,#5112,#5113);
#4690=AXIS2_PLACEMENT_3D('',#5922,#5114,#5115);
#4691=AXIS2_PLACEMENT_3D('',#5926,#5117,#5118);
#4692=AXIS2_PLACEMENT_3D('',#5927,#5119,#5120);
#4693=AXIS2_PLACEMENT_3D('',#5928,#5121,#5122);
#4694=AXIS2_PLACEMENT_3D('',#5933,#5124,#5125);
#4695=AXIS2_PLACEMENT_3D('',#5935,#5127,#5128);
#4696=AXIS2_PLACEMENT_3D('',#5936,#5129,#5130);
#4697=AXIS2_PLACEMENT_3D('',#5940,#5132,#5133);
#4698=AXIS2_PLACEMENT_3D('',#5942,#5135,#5136);
#4699=AXIS2_PLACEMENT_3D('',#5946,#5138,#5139);
#4700=AXIS2_PLACEMENT_3D('',#5948,#5141,#5142);
#4701=AXIS2_PLACEMENT_3D('',#5951,#5144,#5145);
#4702=AXIS2_PLACEMENT_3D('',#5953,#5147,#5148);
#4703=AXIS2_PLACEMENT_3D('',#5956,#5150,#5151);
#4704=AXIS2_PLACEMENT_3D('',#5957,#5152,#5153);
#4705=AXIS2_PLACEMENT_3D('',#5960,#5155,#5156);
#4706=AXIS2_PLACEMENT_3D('',#5961,#5157,#5158);
#4707=AXIS2_PLACEMENT_3D('',#5964,#5160,#5161);
#4708=AXIS2_PLACEMENT_3D('',#5965,#5162,#5163);
#4709=AXIS2_PLACEMENT_3D('',#5967,#5165,#5166);
#4710=AXIS2_PLACEMENT_3D('',#5969,#5168,#5169);
#4711=AXIS2_PLACEMENT_3D('',#5971,#5170,#5171);
#4712=AXIS2_PLACEMENT_3D('',#5973,#5172,#5173);
#4713=AXIS2_PLACEMENT_3D('',#5975,#5174,#5175);
#4714=AXIS2_PLACEMENT_3D('',#5977,#5176,#5177);
#4715=AXIS2_PLACEMENT_3D('',#5979,#5178,#5179);
#4716=AXIS2_PLACEMENT_3D('',#5980,#5180,#5181);
#4717=AXIS2_PLACEMENT_3D('',#5981,#5182,#5183);
#4718=AXIS2_PLACEMENT_3D('',#5982,#5184,#5185);
#4719=AXIS2_PLACEMENT_3D('',#5983,#5186,#5187);
#4720=AXIS2_PLACEMENT_3D('',#5984,#5188,#5189);
#4721=AXIS2_PLACEMENT_3D('',#5985,#5190,#5191);
#4722=AXIS2_PLACEMENT_3D('',#5986,#5192,#5193);
#4723=AXIS2_PLACEMENT_3D('',#5987,#5194,#5195);
#4724=AXIS2_PLACEMENT_3D('',#5988,#5196,#5197);
#4725=AXIS2_PLACEMENT_3D('',#5989,#5198,#5199);
#4726=AXIS2_PLACEMENT_3D('',#5990,#5200,#5201);
#4727=AXIS2_PLACEMENT_3D('',#5992,#5203,#5204);
#4728=AXIS2_PLACEMENT_3D('',#5994,#5206,#5207);
#4949=DIRECTION('axis',(0.,0.,1.));
#4950=DIRECTION('refdir',(1.,0.,0.));
#4951=DIRECTION('center_axis',(0.,0.,1.));
#4952=DIRECTION('ref_axis',(1.,0.,0.));
#4953=DIRECTION('center_axis',(0.,0.,1.));
#4954=DIRECTION('ref_axis',(1.,0.,0.));
#4955=DIRECTION('',(0.,0.,1.));
#4956=DIRECTION('center_axis',(0.,0.,1.));
#4957=DIRECTION('ref_axis',(1.,0.,0.));
#4958=DIRECTION('center_axis',(0.,0.,1.));
#4959=DIRECTION('ref_axis',(1.,0.,0.));
#4960=DIRECTION('center_axis',(0.,0.,-1.));
#4961=DIRECTION('ref_axis',(1.,0.,0.));
#4962=DIRECTION('center_axis',(0.,0.,-1.));
#4963=DIRECTION('ref_axis',(-1.,0.,0.));
#4964=DIRECTION('center_axis',(0.,0.,1.));
#4965=DIRECTION('ref_axis',(1.,0.,0.));
#4966=DIRECTION('center_axis',(0.,0.,1.));
#4967=DIRECTION('ref_axis',(1.,0.,0.));
#4968=DIRECTION('center_axis',(0.,0.,1.));
#4969=DIRECTION('ref_axis',(1.,0.,0.));
#4970=DIRECTION('center_axis',(0.,0.,1.));
#4971=DIRECTION('ref_axis',(1.,0.,0.));
#4972=DIRECTION('',(0.,0.,1.));
#4973=DIRECTION('center_axis',(1.,0.,0.));
#4974=DIRECTION('ref_axis',(0.,0.707106781186546,-0.707106781186549));
#4975=DIRECTION('',(-1.,0.,0.));
#4976=DIRECTION('center_axis',(0.923879532511283,0.382683432365099,3.39891166203453E-15));
#4977=DIRECTION('ref_axis',(-0.382683432365099,0.923879532511283,8.20569863179162E-15));
#4978=DIRECTION('',(1.,0.,0.));
#4979=DIRECTION('center_axis',(0.923879532511286,-0.382683432365092,0.));
#4980=DIRECTION('ref_axis',(0.382683432365092,0.923879532511286,0.));
#4981=DIRECTION('center_axis',(0.707106781186548,0.707106781186548,0.));
#4982=DIRECTION('ref_axis',(-0.5,0.5,-0.707106781186548));
#4983=DIRECTION('',(-0.707106781186547,-0.707106781186547,0.));
#4984=DIRECTION('center_axis',(0.382683432365092,0.923879532511286,0.));
#4985=DIRECTION('ref_axis',(-0.923879532511286,0.382683432365092,0.));
#4986=DIRECTION('',(0.707106781186547,0.707106781186547,0.));
#4987=DIRECTION('center_axis',(0.,1.,0.));
#4988=DIRECTION('ref_axis',(-0.707106781186546,0.,-0.707106781186549));
#4989=DIRECTION('',(0.,-1.,0.));
#4990=DIRECTION('center_axis',(-0.382683432365099,0.923879532511283,3.39891166203453E-15));
#4991=DIRECTION('ref_axis',(-0.923879532511283,-0.382683432365099,8.20569863179162E-15));
#4992=DIRECTION('',(0.,1.,0.));
#4993=DIRECTION('center_axis',(-1.,0.,0.));
#4994=DIRECTION('ref_axis',(0.,-0.707106781186546,-0.707106781186549));
#4995=DIRECTION('',(1.,0.,0.));
#4996=DIRECTION('center_axis',(-0.923879532511283,-0.382683432365099,3.39891166203453E-15));
#4997=DIRECTION('ref_axis',(0.382683432365099,-0.923879532511283,8.20569863179162E-15));
#4998=DIRECTION('',(-1.,0.,0.));
#4999=DIRECTION('center_axis',(0.923879532511286,-0.382683432365092,0.));
#5000=DIRECTION('ref_axis',(0.382683432365092,0.923879532511286,0.));
#5001=DIRECTION('center_axis',(-0.707106781186548,-0.707106781186548,0.));
#5002=DIRECTION('ref_axis',(0.5,-0.5,-0.707106781186548));
#5003=DIRECTION('',(-0.707106781186547,-0.707106781186547,0.));
#5004=DIRECTION('',(0.707106781186547,0.707106781186547,0.));
#5005=DIRECTION('center_axis',(-0.382683432365092,-0.923879532511286,0.));
#5006=DIRECTION('ref_axis',(0.923879532511286,-0.382683432365092,0.));
#5007=DIRECTION('center_axis',(-0.707106781186548,0.707106781186548,0.));
#5008=DIRECTION('ref_axis',(-0.5,-0.5,-0.707106781186548));
#5009=DIRECTION('',(0.707106781186547,-0.707106781186547,0.));
#5010=DIRECTION('',(-0.707106781186547,0.707106781186547,0.));
#5011=DIRECTION('center_axis',(0.,-1.,0.));
#5012=DIRECTION('ref_axis',(0.707106781186546,0.,-0.707106781186549));
#5013=DIRECTION('',(0.,-1.,0.));
#5014=DIRECTION('',(0.,1.,0.));
#5015=DIRECTION('center_axis',(0.382683432365099,-0.923879532511283,3.39891166203453E-15));
#5016=DIRECTION('ref_axis',(0.923879532511283,0.382683432365099,8.20569863179162E-15));
#5017=DIRECTION('center_axis',(0.707106781186548,-0.707106781186548,0.));
#5018=DIRECTION('ref_axis',(0.5,0.5,-0.707106781186548));
#5019=DIRECTION('',(0.707106781186547,-0.707106781186547,0.));
#5020=DIRECTION('',(-0.707106781186547,0.707106781186547,0.));
#5021=DIRECTION('center_axis',(-0.707106781186548,0.707106781186548,0.));
#5022=DIRECTION('ref_axis',(-0.707106781186548,-0.707106781186548,0.));
#5023=DIRECTION('',(0.,0.,1.));
#5024=DIRECTION('',(-0.707106781186547,-0.707106781186547,0.));
#5025=DIRECTION('',(0.,0.,1.));
#5026=DIRECTION('center_axis',(-1.,0.,0.));
#5027=DIRECTION('ref_axis',(0.,-1.,0.));
#5028=DIRECTION('',(0.,0.,1.));
#5029=DIRECTION('',(0.,-1.,0.));
#5030=DIRECTION('center_axis',(-0.707106781186548,-0.707106781186548,0.));
#5031=DIRECTION('ref_axis',(0.707106781186548,-0.707106781186548,0.));
#5032=DIRECTION('',(0.,0.,1.));
#5033=DIRECTION('',(0.707106781186547,-0.707106781186547,0.));
#5034=DIRECTION('center_axis',(0.,-1.,0.));
#5035=DIRECTION('ref_axis',(1.,0.,0.));
#5036=DIRECTION('',(0.,0.,1.));
#5037=DIRECTION('',(1.,0.,0.));
#5038=DIRECTION('center_axis',(0.,0.,1.));
#5039=DIRECTION('ref_axis',(1.,0.,0.));
#5040=DIRECTION('center_axis',(0.,0.,-1.));
#5041=DIRECTION('ref_axis',(1.,0.,0.));
#5042=DIRECTION('center_axis',(0.,0.,-1.));
#5043=DIRECTION('ref_axis',(1.,0.,0.));
#5044=DIRECTION('center_axis',(0.,0.,-1.));
#5045=DIRECTION('ref_axis',(1.,0.,0.));
#5046=DIRECTION('center_axis',(0.,0.,-1.));
#5047=DIRECTION('ref_axis',(1.,0.,0.));
#5048=DIRECTION('center_axis',(0.,0.,-1.));
#5049=DIRECTION('ref_axis',(1.,0.,0.));
#5050=DIRECTION('center_axis',(0.,0.,-1.));
#5051=DIRECTION('ref_axis',(-1.,0.,0.));
#5052=DIRECTION('center_axis',(0.,0.,1.));
#5053=DIRECTION('ref_axis',(1.,0.,0.));
#5054=DIRECTION('center_axis',(0.,-1.,0.));
#5055=DIRECTION('ref_axis',(1.,0.,0.));
#5056=DIRECTION('center_axis',(0.,0.,1.));
#5057=DIRECTION('ref_axis',(1.,0.,0.));
#5058=DIRECTION('center_axis',(0.,0.,1.));
#5059=DIRECTION('ref_axis',(1.,0.,0.));
#5060=DIRECTION('',(0.,0.,1.));
#5061=DIRECTION('center_axis',(0.,0.,-1.));
#5062=DIRECTION('ref_axis',(1.,0.,0.));
#5063=DIRECTION('center_axis',(0.,0.,-1.));
#5064=DIRECTION('ref_axis',(1.,0.,0.));
#5065=DIRECTION('center_axis',(0.,0.,-1.));
#5066=DIRECTION('ref_axis',(-1.,0.,0.));
#5067=DIRECTION('center_axis',(0.,0.,1.));
#5068=DIRECTION('ref_axis',(1.,0.,0.));
#5069=DIRECTION('center_axis',(0.,-1.,0.));
#5070=DIRECTION('ref_axis',(1.,0.,0.));
#5071=DIRECTION('center_axis',(0.,0.,1.));
#5072=DIRECTION('ref_axis',(1.,0.,0.));
#5073=DIRECTION('center_axis',(0.,0.,1.));
#5074=DIRECTION('ref_axis',(1.,0.,0.));
#5075=DIRECTION('',(0.,0.,1.));
#5076=DIRECTION('center_axis',(0.,0.,-1.));
#5077=DIRECTION('ref_axis',(1.,0.,0.));
#5078=DIRECTION('center_axis',(0.,0.,-1.));
#5079=DIRECTION('ref_axis',(1.,0.,0.));
#5080=DIRECTION('center_axis',(0.,0.,-1.));
#5081=DIRECTION('ref_axis',(-1.,0.,0.));
#5082=DIRECTION('center_axis',(0.,0.,1.));
#5083=DIRECTION('ref_axis',(1.,0.,0.));
#5084=DIRECTION('center_axis',(0.,-1.,0.));
#5085=DIRECTION('ref_axis',(1.,0.,0.));
#5086=DIRECTION('center_axis',(0.,0.,1.));
#5087=DIRECTION('ref_axis',(1.,0.,0.));
#5088=DIRECTION('center_axis',(0.,0.,1.));
#5089=DIRECTION('ref_axis',(1.,0.,0.));
#5090=DIRECTION('',(0.,0.,1.));
#5091=DIRECTION('center_axis',(0.,0.,-1.));
#5092=DIRECTION('ref_axis',(1.,0.,0.));
#5093=DIRECTION('center_axis',(0.,0.,-1.));
#5094=DIRECTION('ref_axis',(1.,0.,0.));
#5095=DIRECTION('center_axis',(0.,0.,-1.));
#5096=DIRECTION('ref_axis',(-1.,0.,0.));
#5097=DIRECTION('center_axis',(-1.22464679914735E-16,-1.,0.));
#5098=DIRECTION('ref_axis',(1.,-1.22464679914735E-16,0.));
#5099=DIRECTION('center_axis',(0.,0.,1.));
#5100=DIRECTION('ref_axis',(1.,0.,0.));
#5101=DIRECTION('',(0.,0.,1.));
#5102=DIRECTION('center_axis',(0.,0.,-1.));
#5103=DIRECTION('ref_axis',(1.,0.,0.));
#5104=DIRECTION('center_axis',(0.,0.,-1.));
#5105=DIRECTION('ref_axis',(1.,0.,0.));
#5106=DIRECTION('center_axis',(0.,0.,-1.));
#5107=DIRECTION('ref_axis',(-1.,0.,0.));
#5108=DIRECTION('center_axis',(0.,0.,1.));
#5109=DIRECTION('ref_axis',(1.,0.,0.));
#5110=DIRECTION('center_axis',(0.,-1.,0.));
#5111=DIRECTION('ref_axis',(1.,0.,0.));
#5112=DIRECTION('center_axis',(0.,0.,1.));
#5113=DIRECTION('ref_axis',(1.,0.,0.));
#5114=DIRECTION('center_axis',(0.,0.,1.));
#5115=DIRECTION('ref_axis',(1.,0.,0.));
#5116=DIRECTION('',(0.,0.,1.));
#5117=DIRECTION('center_axis',(0.,0.,-1.));
#5118=DIRECTION('ref_axis',(1.,0.,0.));
#5119=DIRECTION('center_axis',(0.,0.,-1.));
#5120=DIRECTION('ref_axis',(1.,0.,0.));
#5121=DIRECTION('center_axis',(-1.,0.,0.));
#5122=DIRECTION('ref_axis',(0.,0.707106781186546,0.707106781186549));
#5123=DIRECTION('',(1.,0.,0.));
#5124=DIRECTION('center_axis',(-0.923879532511286,0.382683432365092,0.));
#5125=DIRECTION('ref_axis',(0.382683432365092,0.923879532511286,0.));
#5126=DIRECTION('',(-1.,0.,0.));
#5127=DIRECTION('center_axis',(-0.923879532511286,-0.382683432365092,8.20569863179164E-15));
#5128=DIRECTION('ref_axis',(-0.382683432365092,0.923879532511286,1.98103089256178E-14));
#5129=DIRECTION('center_axis',(-0.707106781186548,0.707106781186548,0.));
#5130=DIRECTION('ref_axis',(0.499999999999999,0.499999999999999,0.707106781186549));
#5131=DIRECTION('',(0.707106781186547,-0.707106781186547,0.));
#5132=DIRECTION('center_axis',(-0.382683432365092,0.923879532511286,8.20569863179164E-15));
#5133=DIRECTION('ref_axis',(0.923879532511286,0.382683432365092,1.98103089256178E-14));
#5134=DIRECTION('',(-0.707106781186547,0.707106781186547,0.));
#5135=DIRECTION('center_axis',(0.,1.,0.));
#5136=DIRECTION('ref_axis',(0.707106781186546,0.,0.707106781186549));
#5137=DIRECTION('',(0.,-1.,0.));
#5138=DIRECTION('center_axis',(0.382683432365092,0.923879532511286,0.));
#5139=DIRECTION('ref_axis',(0.923879532511286,-0.382683432365092,0.));
#5140=DIRECTION('',(0.,1.,0.));
#5141=DIRECTION('center_axis',(0.707106781186548,0.707106781186548,0.));
#5142=DIRECTION('ref_axis',(0.499999999999999,-0.499999999999999,0.707106781186549));
#5143=DIRECTION('',(-0.707106781186547,-0.707106781186547,0.));
#5144=DIRECTION('center_axis',(0.923879532511286,0.382683432365092,8.20569863179164E-15));
#5145=DIRECTION('ref_axis',(0.382683432365092,-0.923879532511286,1.98103089256178E-14));
#5146=DIRECTION('',(0.707106781186547,0.707106781186547,0.));
#5147=DIRECTION('center_axis',(1.,0.,0.));
#5148=DIRECTION('ref_axis',(0.,-0.707106781186546,0.707106781186549));
#5149=DIRECTION('',(-1.,0.,0.));
#5150=DIRECTION('center_axis',(0.923879532511286,-0.382683432365092,0.));
#5151=DIRECTION('ref_axis',(-0.382683432365092,-0.923879532511286,0.));
#5152=DIRECTION('center_axis',(0.707106781186548,-0.707106781186548,0.));
#5153=DIRECTION('ref_axis',(-0.499999999999999,-0.499999999999999,0.707106781186549));
#5154=DIRECTION('',(-0.707106781186547,0.707106781186547,0.));
#5155=DIRECTION('center_axis',(0.382683432365092,-0.923879532511286,8.20569863179164E-15));
#5156=DIRECTION('ref_axis',(-0.923879532511286,-0.382683432365092,1.98103089256178E-14));
#5157=DIRECTION('center_axis',(0.,-1.,0.));
#5158=DIRECTION('ref_axis',(-0.707106781186546,0.,0.707106781186549));
#5159=DIRECTION('',(0.,1.,0.));
#5160=DIRECTION('center_axis',(-0.382683432365092,-0.923879532511286,0.));
#5161=DIRECTION('ref_axis',(-0.923879532511286,0.382683432365092,0.));
#5162=DIRECTION('center_axis',(-0.707106781186548,-0.707106781186548,0.));
#5163=DIRECTION('ref_axis',(-0.499999999999999,0.499999999999999,0.707106781186549));
#5164=DIRECTION('',(0.707106781186547,0.707106781186547,0.));
#5165=DIRECTION('center_axis',(0.,1.,0.));
#5166=DIRECTION('ref_axis',(-1.,0.,0.));
#5167=DIRECTION('',(0.,0.,1.));
#5168=DIRECTION('center_axis',(0.,0.,1.));
#5169=DIRECTION('ref_axis',(1.,0.,0.));
#5170=DIRECTION('center_axis',(0.,0.,1.));
#5171=DIRECTION('ref_axis',(1.,0.,0.));
#5172=DIRECTION('center_axis',(0.,0.,1.));
#5173=DIRECTION('ref_axis',(1.,0.,0.));
#5174=DIRECTION('center_axis',(0.,0.,1.));
#5175=DIRECTION('ref_axis',(1.,0.,0.));
#5176=DIRECTION('center_axis',(0.,0.,1.));
#5177=DIRECTION('ref_axis',(1.,0.,0.));
#5178=DIRECTION('center_axis',(0.,0.,1.));
#5179=DIRECTION('ref_axis',(1.,0.,0.));
#5180=DIRECTION('center_axis',(0.,0.,-1.));
#5181=DIRECTION('ref_axis',(-1.,0.,0.));
#5182=DIRECTION('center_axis',(0.,-1.,0.));
#5183=DIRECTION('ref_axis',(1.,0.,0.));
#5184=DIRECTION('center_axis',(0.,0.,-1.));
#5185=DIRECTION('ref_axis',(-1.,0.,0.));
#5186=DIRECTION('center_axis',(0.,-1.,0.));
#5187=DIRECTION('ref_axis',(1.,0.,0.));
#5188=DIRECTION('center_axis',(0.,0.,-1.));
#5189=DIRECTION('ref_axis',(-1.,0.,0.));
#5190=DIRECTION('center_axis',(0.,-1.,0.));
#5191=DIRECTION('ref_axis',(1.,0.,0.));
#5192=DIRECTION('center_axis',(0.,0.,-1.));
#5193=DIRECTION('ref_axis',(-1.,0.,0.));
#5194=DIRECTION('center_axis',(-1.22464679914735E-16,-1.,0.));
#5195=DIRECTION('ref_axis',(1.,-1.22464679914735E-16,0.));
#5196=DIRECTION('center_axis',(0.,0.,-1.));
#5197=DIRECTION('ref_axis',(-1.,0.,0.));
#5198=DIRECTION('center_axis',(0.,-1.,0.));
#5199=DIRECTION('ref_axis',(1.,0.,0.));
#5200=DIRECTION('center_axis',(0.707106781186548,0.707106781186548,0.));
#5201=DIRECTION('ref_axis',(-0.707106781186548,0.707106781186548,0.));
#5202=DIRECTION('',(0.,0.,1.));
#5203=DIRECTION('center_axis',(1.,0.,0.));
#5204=DIRECTION('ref_axis',(0.,1.,0.));
#5205=DIRECTION('',(0.,0.,1.));
#5206=DIRECTION('center_axis',(0.707106781186548,-0.707106781186548,0.));
#5207=DIRECTION('ref_axis',(0.707106781186548,0.707106781186548,0.));
#5776=CARTESIAN_POINT('',(0.,0.,0.));
#5777=CARTESIAN_POINT('Origin',(0.,0.,4.));
#5778=CARTESIAN_POINT('',(-20.5,-2.51052593825207E-15,2.06740544556191));
#5779=CARTESIAN_POINT('Origin',(0.,0.,2.06740544556191));
#5780=CARTESIAN_POINT('',(-20.5,-2.51052593825207E-15,5.93259455443809));
#5781=CARTESIAN_POINT('',(-20.5,-2.51052593825207E-15,4.));
#5782=CARTESIAN_POINT('Origin',(0.,0.,5.93259455443809));
#5783=CARTESIAN_POINT('Origin',(19.5,0.,5.93259455443809));
#5784=CARTESIAN_POINT('',(-20.,2.44929359829471E-15,5.93259455443809));
#5785=CARTESIAN_POINT('Origin',(0.,0.,5.93259455443809));
#5786=CARTESIAN_POINT('Origin',(20.5,0.,2.06740544556191));
#5787=CARTESIAN_POINT('',(-20.,-2.44929359829471E-15,2.06740544556191));
#5788=CARTESIAN_POINT('Origin',(0.,0.,2.06740544556191));
#5789=CARTESIAN_POINT('Origin',(0.,0.,0.));
#5790=CARTESIAN_POINT('',(20.,-2.44929359829471E-15,0.5));
#5791=CARTESIAN_POINT('',(-20.,-2.44929359829471E-15,0.5));
#5792=CARTESIAN_POINT('Origin',(0.,0.,0.5));
#5793=CARTESIAN_POINT('Origin',(0.,0.,0.5));
#5794=CARTESIAN_POINT('',(-20.,-2.44929359829471E-15,0.));
#5795=CARTESIAN_POINT('Origin',(13.5,29.5,0.5));
#5796=CARTESIAN_POINT('',(26.7928932188135,29.5,0.));
#5797=CARTESIAN_POINT('',(-26.7928932188135,29.5,0.));
#5798=CARTESIAN_POINT('',(13.5,29.5,0.));
#5799=CARTESIAN_POINT('',(-27.,30.,0.5));
#5800=CARTESIAN_POINT('Origin',(-26.7928932188135,29.5,0.5));
#5801=CARTESIAN_POINT('',(27.,30.,0.5));
#5802=CARTESIAN_POINT('',(13.5,30.,0.5));
#5803=CARTESIAN_POINT('Origin',(26.7928932188135,29.5,0.5));
#5804=CARTESIAN_POINT('Origin',(-27.3964466094067,28.8964466094067,0.5));
#5805=CARTESIAN_POINT('',(-29.5,26.7928932188135,0.));
#5806=CARTESIAN_POINT('',(-27.3964466094067,28.8964466094067,0.));
#5807=CARTESIAN_POINT('',(-30.,27.,0.5));
#5808=CARTESIAN_POINT('Origin',(-29.5,26.7928932188135,0.5));
#5809=CARTESIAN_POINT('',(-27.75,29.25,0.5));
#5810=CARTESIAN_POINT('Origin',(-29.5,13.5,0.5));
#5811=CARTESIAN_POINT('',(-29.5,-26.7928932188135,0.));
#5812=CARTESIAN_POINT('',(-29.5,13.5,0.));
#5813=CARTESIAN_POINT('',(-30.,-27.,0.5));
#5814=CARTESIAN_POINT('Origin',(-29.5,-26.7928932188135,0.5));
#5815=CARTESIAN_POINT('',(-30.,13.5,0.5));
#5816=CARTESIAN_POINT('Origin',(-13.5,-29.5,0.5));
#5817=CARTESIAN_POINT('',(-26.7928932188135,-29.5,0.));
#5818=CARTESIAN_POINT('',(26.7928932188135,-29.5,0.));
#5819=CARTESIAN_POINT('',(-13.5,-29.5,0.));
#5820=CARTESIAN_POINT('',(27.,-30.,0.5));
#5821=CARTESIAN_POINT('Origin',(26.7928932188135,-29.5,0.5));
#5822=CARTESIAN_POINT('',(-27.,-30.,0.5));
#5823=CARTESIAN_POINT('',(-13.5,-30.,0.5));
#5824=CARTESIAN_POINT('Origin',(-26.7928932188135,-29.5,0.5));
#5825=CARTESIAN_POINT('Origin',(27.3964466094067,-28.8964466094067,0.5));
#5826=CARTESIAN_POINT('',(30.,-27.,0.5));
#5827=CARTESIAN_POINT('',(27.75,-29.25,0.5));
#5828=CARTESIAN_POINT('',(29.5,-26.7928932188135,0.));
#5829=CARTESIAN_POINT('',(27.3964466094067,-28.8964466094067,0.));
#5830=CARTESIAN_POINT('Origin',(29.5,-26.7928932188135,0.5));
#5831=CARTESIAN_POINT('Origin',(-28.8964466094067,-27.3964466094067,0.5));
#5832=CARTESIAN_POINT('',(-28.8964466094067,-27.3964466094067,0.));
#5833=CARTESIAN_POINT('',(-29.25,-27.75,0.5));
#5834=CARTESIAN_POINT('Origin',(29.5,-13.5,0.5));
#5835=CARTESIAN_POINT('',(30.,27.,0.5));
#5836=CARTESIAN_POINT('',(30.,-13.5,0.5));
#5837=CARTESIAN_POINT('',(29.5,26.7928932188135,0.));
#5838=CARTESIAN_POINT('',(29.5,-13.5,0.));
#5839=CARTESIAN_POINT('Origin',(29.5,26.7928932188135,0.5));
#5840=CARTESIAN_POINT('Origin',(28.8964466094067,27.3964466094067,0.5));
#5841=CARTESIAN_POINT('',(29.25,27.75,0.5));
#5842=CARTESIAN_POINT('',(28.8964466094067,27.3964466094067,0.));
#5843=CARTESIAN_POINT('Origin',(-27.,30.,0.));
#5844=CARTESIAN_POINT('',(-30.,27.,7.5));
#5845=CARTESIAN_POINT('',(-30.,27.,0.));
#5846=CARTESIAN_POINT('',(-27.,30.,7.5));
#5847=CARTESIAN_POINT('',(-27.75,29.25,7.5));
#5848=CARTESIAN_POINT('',(-27.,30.,0.));
#5849=CARTESIAN_POINT('Origin',(-30.,27.,0.));
#5850=CARTESIAN_POINT('',(-30.,-27.,7.5));
#5851=CARTESIAN_POINT('',(-30.,-27.,0.));
#5852=CARTESIAN_POINT('',(-30.,13.5,7.5));
#5853=CARTESIAN_POINT('Origin',(-30.,-27.,0.));
#5854=CARTESIAN_POINT('',(-27.,-30.,7.5));
#5855=CARTESIAN_POINT('',(-27.,-30.,0.));
#5856=CARTESIAN_POINT('',(-29.25,-27.75,7.5));
#5857=CARTESIAN_POINT('Origin',(-27.,-30.,0.));
#5858=CARTESIAN_POINT('',(27.,-30.,7.5));
#5859=CARTESIAN_POINT('',(27.,-30.,0.));
#5860=CARTESIAN_POINT('',(-13.5,-30.,7.5));
#5861=CARTESIAN_POINT('Origin',(0.,0.,0.));
#5862=CARTESIAN_POINT('',(28.0502525316942,-23.5502525316942,0.));
#5863=CARTESIAN_POINT('Origin',(23.5502525316942,-23.5502525316942,0.));
#5864=CARTESIAN_POINT('',(-19.0502525316942,23.5502525316942,0.));
#5865=CARTESIAN_POINT('Origin',(-23.5502525316942,23.5502525316942,0.));
#5866=CARTESIAN_POINT('',(-19.0502525316942,-23.5502525316942,0.));
#5867=CARTESIAN_POINT('Origin',(-23.5502525316942,-23.5502525316942,0.));
#5868=CARTESIAN_POINT('',(20.5,-2.51052593825207E-15,0.));
#5869=CARTESIAN_POINT('Origin',(0.,0.,0.));
#5870=CARTESIAN_POINT('',(28.0502525316942,23.5502525316942,0.));
#5871=CARTESIAN_POINT('Origin',(23.5502525316942,23.5502525316942,0.));
#5872=CARTESIAN_POINT('Origin',(23.5502525316942,-23.5502525316942,0.5));
#5873=CARTESIAN_POINT('',(19.5502525316942,-23.5502525316942,0.5));
#5874=CARTESIAN_POINT('',(27.5502525316942,-23.5502525316942,0.5));
#5875=CARTESIAN_POINT('Origin',(23.5502525316942,-23.5502525316942,0.5));
#5876=CARTESIAN_POINT('Origin',(28.0502525316942,-23.5502525316942,0.5));
#5877=CARTESIAN_POINT('Origin',(23.5502525316942,-23.5502525316942,0.5));
#5878=CARTESIAN_POINT('Origin',(23.5502525316942,-23.5502525316942,0.));
#5879=CARTESIAN_POINT('',(19.5502525316942,-23.5502525316942,7.5));
#5880=CARTESIAN_POINT('',(19.5502525316942,-23.5502525316942,0.));
#5881=CARTESIAN_POINT('',(27.5502525316942,-23.5502525316942,7.5));
#5882=CARTESIAN_POINT('Origin',(23.5502525316942,-23.5502525316942,7.5));
#5883=CARTESIAN_POINT('Origin',(23.5502525316942,-23.5502525316942,7.5));
#5884=CARTESIAN_POINT('Origin',(23.5502525316942,23.5502525316942,0.5));
#5885=CARTESIAN_POINT('',(19.5502525316942,23.5502525316942,0.5));
#5886=CARTESIAN_POINT('',(27.5502525316942,23.5502525316942,0.5));
#5887=CARTESIAN_POINT('Origin',(23.5502525316942,23.5502525316942,0.5));
#5888=CARTESIAN_POINT('Origin',(28.0502525316942,23.5502525316942,0.5));
#5889=CARTESIAN_POINT('Origin',(23.5502525316942,23.5502525316942,0.5));
#5890=CARTESIAN_POINT('Origin',(23.5502525316942,23.5502525316942,0.));
#5891=CARTESIAN_POINT('',(19.5502525316942,23.5502525316942,7.5));
#5892=CARTESIAN_POINT('',(19.5502525316942,23.5502525316942,0.));
#5893=CARTESIAN_POINT('',(27.5502525316942,23.5502525316942,7.5));
#5894=CARTESIAN_POINT('Origin',(23.5502525316942,23.5502525316942,7.5));
#5895=CARTESIAN_POINT('Origin',(23.5502525316942,23.5502525316942,7.5));
#5896=CARTESIAN_POINT('Origin',(-23.5502525316942,23.5502525316942,0.5));
#5897=CARTESIAN_POINT('',(-27.5502525316942,23.5502525316942,0.5));
#5898=CARTESIAN_POINT('',(-19.5502525316942,23.5502525316942,0.5));
#5899=CARTESIAN_POINT('Origin',(-23.5502525316942,23.5502525316942,0.5));
#5900=CARTESIAN_POINT('Origin',(-19.0502525316942,23.5502525316942,0.5));
#5901=CARTESIAN_POINT('Origin',(-23.5502525316942,23.5502525316942,0.5));
#5902=CARTESIAN_POINT('Origin',(-23.5502525316942,23.5502525316942,0.));
#5903=CARTESIAN_POINT('',(-27.5502525316942,23.5502525316942,7.5));
#5904=CARTESIAN_POINT('',(-27.5502525316942,23.5502525316942,0.));
#5905=CARTESIAN_POINT('',(-19.5502525316942,23.5502525316942,7.5));
#5906=CARTESIAN_POINT('Origin',(-23.5502525316942,23.5502525316942,7.5));
#5907=CARTESIAN_POINT('Origin',(-23.5502525316942,23.5502525316942,7.5));
#5908=CARTESIAN_POINT('Origin',(0.,0.,0.5));
#5909=CARTESIAN_POINT('Origin',(20.5,-2.51052593825207E-15,0.5));
#5910=CARTESIAN_POINT('Origin',(0.,0.,0.));
#5911=CARTESIAN_POINT('',(-20.,-2.44929359829471E-15,7.5));
#5912=CARTESIAN_POINT('',(-20.,-2.44929359829471E-15,0.));
#5913=CARTESIAN_POINT('',(20.,-2.44929359829471E-15,7.5));
#5914=CARTESIAN_POINT('Origin',(0.,0.,7.5));
#5915=CARTESIAN_POINT('Origin',(0.,0.,7.5));
#5916=CARTESIAN_POINT('Origin',(-23.5502525316942,-23.5502525316942,0.5));
#5917=CARTESIAN_POINT('',(-27.5502525316942,-23.5502525316942,0.5));
#5918=CARTESIAN_POINT('',(-19.5502525316942,-23.5502525316942,0.5));
#5919=CARTESIAN_POINT('Origin',(-23.5502525316942,-23.5502525316942,0.5));
#5920=CARTESIAN_POINT('Origin',(-19.0502525316942,-23.5502525316942,0.5));
#5921=CARTESIAN_POINT('Origin',(-23.5502525316942,-23.5502525316942,0.5));
#5922=CARTESIAN_POINT('Origin',(-23.5502525316942,-23.5502525316942,0.));
#5923=CARTESIAN_POINT('',(-27.5502525316942,-23.5502525316942,7.5));
#5924=CARTESIAN_POINT('',(-27.5502525316942,-23.5502525316942,0.));
#5925=CARTESIAN_POINT('',(-19.5502525316942,-23.5502525316942,7.5));
#5926=CARTESIAN_POINT('Origin',(-23.5502525316942,-23.5502525316942,7.5));
#5927=CARTESIAN_POINT('Origin',(-23.5502525316942,-23.5502525316942,7.5));
#5928=CARTESIAN_POINT('Origin',(13.5,29.5,7.5));
#5929=CARTESIAN_POINT('',(-26.7928932188135,29.5,8.));
#5930=CARTESIAN_POINT('',(26.7928932188135,29.5,8.));
#5931=CARTESIAN_POINT('',(13.5,29.5,8.));
#5932=CARTESIAN_POINT('',(27.,30.,7.5));
#5933=CARTESIAN_POINT('Origin',(26.7928932188135,29.5,7.5));
#5934=CARTESIAN_POINT('',(13.5,30.,7.5));
#5935=CARTESIAN_POINT('Origin',(-26.7928932188135,29.5,7.5));
#5936=CARTESIAN_POINT('Origin',(28.8964466094067,27.3964466094067,7.5));
#5937=CARTESIAN_POINT('',(29.5,26.7928932188135,8.));
#5938=CARTESIAN_POINT('',(28.8964466094067,27.3964466094067,8.));
#5939=CARTESIAN_POINT('',(30.,27.,7.5));
#5940=CARTESIAN_POINT('Origin',(29.5,26.7928932188135,7.5));
#5941=CARTESIAN_POINT('',(29.25,27.75,7.5));
#5942=CARTESIAN_POINT('Origin',(29.5,-13.5,7.5));
#5943=CARTESIAN_POINT('',(29.5,-26.7928932188135,8.));
#5944=CARTESIAN_POINT('',(29.5,-13.5,8.));
#5945=CARTESIAN_POINT('',(30.,-27.,7.5));
#5946=CARTESIAN_POINT('Origin',(29.5,-26.7928932188135,7.5));
#5947=CARTESIAN_POINT('',(30.,-13.5,7.5));
#5948=CARTESIAN_POINT('Origin',(27.3964466094067,-28.8964466094067,7.5));
#5949=CARTESIAN_POINT('',(26.7928932188135,-29.5,8.));
#5950=CARTESIAN_POINT('',(27.3964466094067,-28.8964466094067,8.));
#5951=CARTESIAN_POINT('Origin',(26.7928932188135,-29.5,7.5));
#5952=CARTESIAN_POINT('',(27.75,-29.25,7.5));
#5953=CARTESIAN_POINT('Origin',(-13.5,-29.5,7.5));
#5954=CARTESIAN_POINT('',(-26.7928932188135,-29.5,8.));
#5955=CARTESIAN_POINT('',(-13.5,-29.5,8.));
#5956=CARTESIAN_POINT('Origin',(-26.7928932188135,-29.5,7.5));
#5957=CARTESIAN_POINT('Origin',(-28.8964466094067,-27.3964466094067,7.5));
#5958=CARTESIAN_POINT('',(-29.5,-26.7928932188135,8.));
#5959=CARTESIAN_POINT('',(-28.8964466094067,-27.3964466094067,8.));
#5960=CARTESIAN_POINT('Origin',(-29.5,-26.7928932188135,7.5));
#5961=CARTESIAN_POINT('Origin',(-29.5,13.5,7.5));
#5962=CARTESIAN_POINT('',(-29.5,26.7928932188135,8.));
#5963=CARTESIAN_POINT('',(-29.5,13.5,8.));
#5964=CARTESIAN_POINT('Origin',(-29.5,26.7928932188135,7.5));
#5965=CARTESIAN_POINT('Origin',(-27.3964466094067,28.8964466094067,7.5));
#5966=CARTESIAN_POINT('',(-27.3964466094067,28.8964466094067,8.));
#5967=CARTESIAN_POINT('Origin',(27.,30.,0.));
#5968=CARTESIAN_POINT('',(27.,30.,0.));
#5969=CARTESIAN_POINT('Origin',(0.,0.,8.));
#5970=CARTESIAN_POINT('',(28.0502525316942,-23.5502525316942,8.));
#5971=CARTESIAN_POINT('Origin',(23.5502525316942,-23.5502525316942,8.));
#5972=CARTESIAN_POINT('',(-19.0502525316942,23.5502525316942,8.));
#5973=CARTESIAN_POINT('Origin',(-23.5502525316942,23.5502525316942,8.));
#5974=CARTESIAN_POINT('',(-19.0502525316942,-23.5502525316942,8.));
#5975=CARTESIAN_POINT('Origin',(-23.5502525316942,-23.5502525316942,8.));
#5976=CARTESIAN_POINT('',(20.5,-2.51052593825207E-15,8.));
#5977=CARTESIAN_POINT('Origin',(0.,0.,8.));
#5978=CARTESIAN_POINT('',(28.0502525316942,23.5502525316942,8.));
#5979=CARTESIAN_POINT('Origin',(23.5502525316942,23.5502525316942,8.));
#5980=CARTESIAN_POINT('Origin',(23.5502525316942,-23.5502525316942,7.5));
#5981=CARTESIAN_POINT('Origin',(28.0502525316942,-23.5502525316942,7.5));
#5982=CARTESIAN_POINT('Origin',(23.5502525316942,23.5502525316942,7.5));
#5983=CARTESIAN_POINT('Origin',(28.0502525316942,23.5502525316942,7.5));
#5984=CARTESIAN_POINT('Origin',(-23.5502525316942,23.5502525316942,7.5));
#5985=CARTESIAN_POINT('Origin',(-19.0502525316942,23.5502525316942,7.5));
#5986=CARTESIAN_POINT('Origin',(0.,0.,7.5));
#5987=CARTESIAN_POINT('Origin',(20.5,-2.51052593825207E-15,7.5));
#5988=CARTESIAN_POINT('Origin',(-23.5502525316942,-23.5502525316942,7.5));
#5989=CARTESIAN_POINT('Origin',(-19.0502525316942,-23.5502525316942,7.5));
#5990=CARTESIAN_POINT('Origin',(30.,27.,0.));
#5991=CARTESIAN_POINT('',(30.,27.,0.));
#5992=CARTESIAN_POINT('Origin',(30.,-27.,0.));
#5993=CARTESIAN_POINT('',(30.,-27.,0.));
#5994=CARTESIAN_POINT('Origin',(27.,-30.,0.));
#74093=UNCERTAINTY_MEASURE_WITH_UNIT(LENGTH_MEASURE(0.01),#74104,
'DISTANCE_ACCURACY_VALUE',
'Maximum model space distance between geometric entities at asserted c
onnectivities');
#74097=UNCERTAINTY_MEASURE_WITH_UNIT(LENGTH_MEASURE(0.01),#74104,
'DISTANCE_ACCURACY_VALUE',
'Maximum model space distance between geometric entities at asserted c
onnectivities');
#74099=(
GEOMETRIC_REPRESENTATION_CONTEXT(3)
GLOBAL_UNCERTAINTY_ASSIGNED_CONTEXT((#74093))
GLOBAL_UNIT_ASSIGNED_CONTEXT((#74104,#74106,#74107))
REPRESENTATION_CONTEXT('','3D')
);
#74103=(
GEOMETRIC_REPRESENTATION_CONTEXT(3)
GLOBAL_UNCERTAINTY_ASSIGNED_CONTEXT((#74097))
GLOBAL_UNIT_ASSIGNED_CONTEXT((#74104,#74106,#74107))
REPRESENTATION_CONTEXT('','3D')
);
#74104=(
LENGTH_UNIT()
NAMED_UNIT(*)
SI_UNIT(.MILLI.,.METRE.)
);
#74106=(
NAMED_UNIT(*)
PLANE_ANGLE_UNIT()
SI_UNIT($,.RADIAN.)
);
#74107=(
NAMED_UNIT(*)
SI_UNIT($,.STERADIAN.)
SOLID_ANGLE_UNIT()
);
#74109=SHAPE_DEFINITION_REPRESENTATION(#74114,#74128);
#74114=PRODUCT_DEFINITION_SHAPE('',$,#74134);
#74128=SHAPE_REPRESENTATION('',(#4623),#74099);
#74132=PRODUCT_DEFINITION_CONTEXT('part definition',#74149,'design');
#74134=PRODUCT_DEFINITION('Top_Part','Top_Part',#74139,#74132);
#74139=PRODUCT_DEFINITION_FORMATION('',$,#74152);
#74149=APPLICATION_CONTEXT(
'Core Data for Automotive Mechanical Design Process');
#74150=PRODUCT_CONTEXT('part definition',#74149,'mechanical');
#74152=PRODUCT('Top_Part','Top_Part',$,(#74150));
#74157=PRESENTATION_STYLE_ASSIGNMENT((#74161));
#74161=SURFACE_STYLE_USAGE(.BOTH.,#74165);
#74165=SURFACE_SIDE_STYLE('',(#74169));
#74169=SURFACE_STYLE_FILL_AREA(#74173);
#74173=FILL_AREA_STYLE('Opaque(55,55,55)',(#74177));
#74177=FILL_AREA_STYLE_COLOUR('Opaque(55,55,55)',#74181);
#74181=COLOUR_RGB('Opaque(55,55,55)', 0.09019608, 0.27058824, 0.51372549);
ENDSEC;
END-ISO-10303-21;
